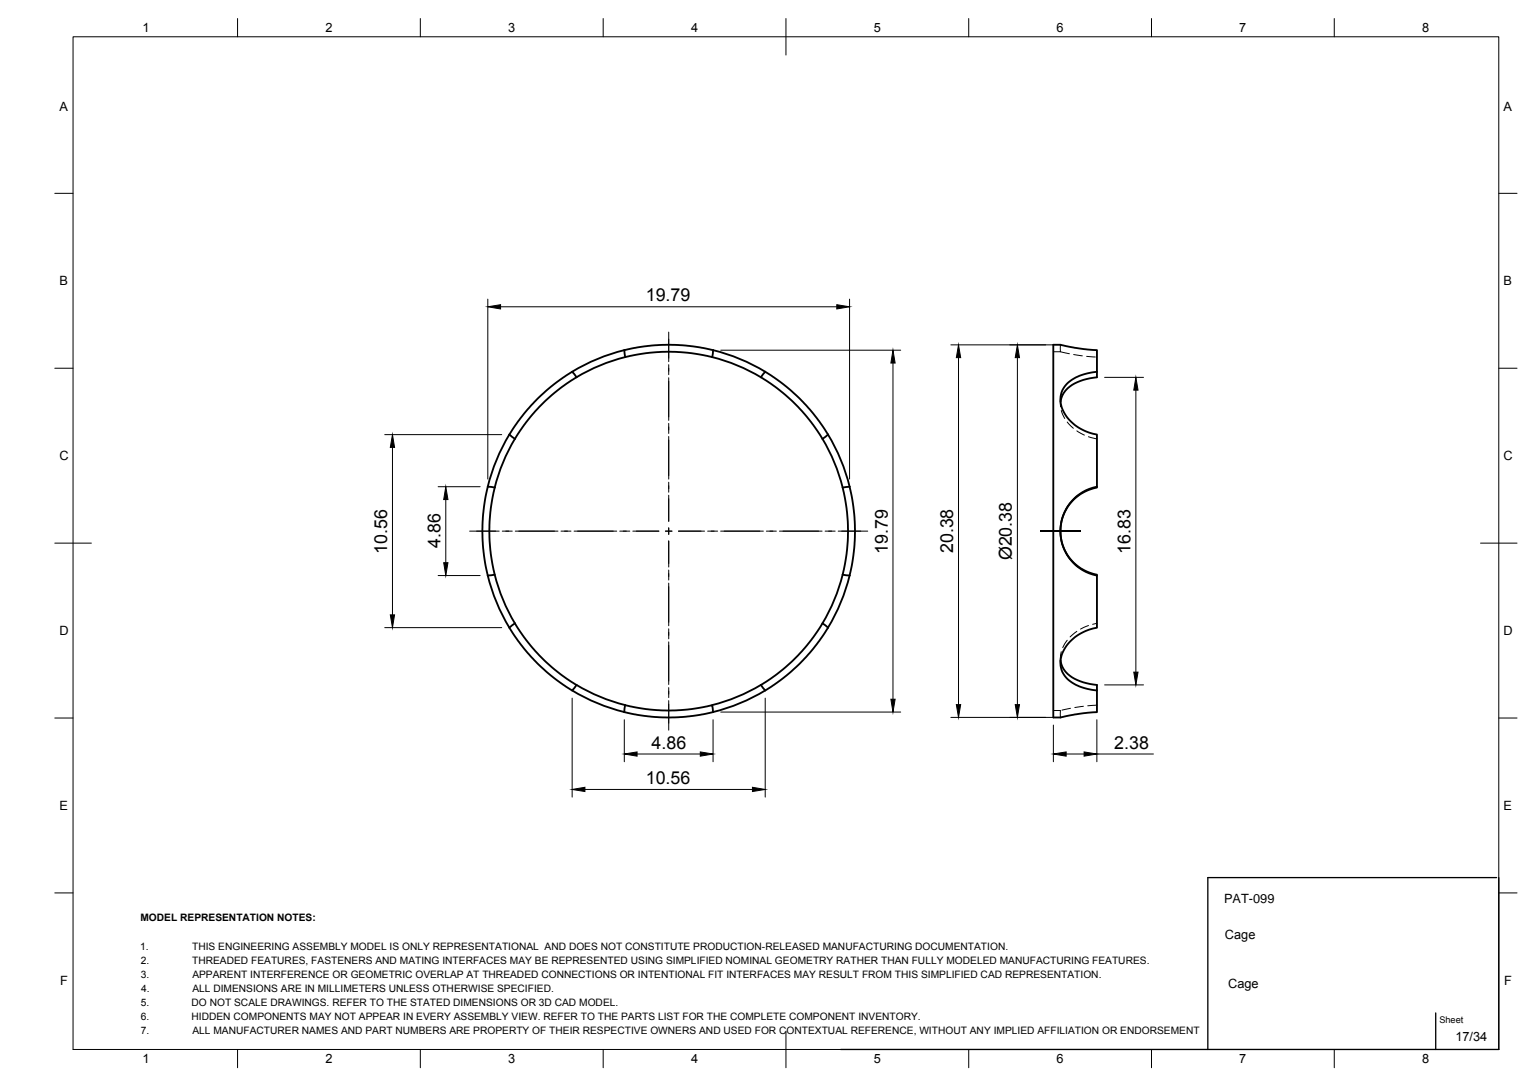
ISO-10303-21;
HEADER;
/* Generated by software containing ST-Developer
 * from STEP Tools, Inc. (www.steptools.com) 
 */

FILE_DESCRIPTION(
/* description */ ('PAT-099'),
/* implementation_level */ '2;1');

FILE_NAME(
/* name */ 'Cage.step',
/* time_stamp */ '2026-10-29T17:25:42-07:00',
/* author */ (''),
/* organization */ (''),
/* preprocessor_version */ 'ST-DEVELOPER v20.2',
/* originating_system */ 'Autodesk Translation Framework v15.17.0.0',
/* authorisation */ '');

FILE_SCHEMA (('AUTOMOTIVE_DESIGN { 1 0 10303 214 3 1 1 }'));
ENDSEC;

DATA;
#10=MECHANICAL_DESIGN_GEOMETRIC_PRESENTATION_REPRESENTATION('',(#367),#11035);
#19=SPHERICAL_SURFACE('',#5561,0.247676);
#20=SPHERICAL_SURFACE('',#5577,0.247676);
#21=SPHERICAL_SURFACE('',#5582,0.247676);
#22=SPHERICAL_SURFACE('',#5587,0.247676);
#23=SPHERICAL_SURFACE('',#5592,0.247676);
#24=SPHERICAL_SURFACE('',#5597,0.247676);
#25=SPHERICAL_SURFACE('',#5602,0.247676);
#26=SPHERICAL_SURFACE('',#5610,0.247676);
#269=B_SPLINE_CURVE_WITH_KNOTS('',3,(#10460,#10461,#10462,#10463,#10464,
#10465,#10466,#10467,#10468,#10469,#10470,#10471,#10472,#10473,#10474,#10475,
#10476,#10477,#10478,#10479,#10480,#10481),.UNSPECIFIED.,.F.,.F.,(4,2,2,
2,2,2,2,2,2,2,4),(0.0473477652366656,0.126350602536658,0.189525903804987,
0.252701205073317,0.313298422430275,0.373895639787233,0.434492857144191,
0.495090074501149,0.558265375769478,0.621440677037807,0.7004435143378),
 .UNSPECIFIED.);
#270=B_SPLINE_CURVE_WITH_KNOTS('',3,(#10485,#10486,#10487,#10488,#10489,
#10490,#10491,#10492,#10493,#10494,#10495,#10496,#10497,#10498,#10499,#10500,
#10501,#10502,#10503,#10504,#10505,#10506),.UNSPECIFIED.,.F.,.F.,(4,2,2,
2,2,2,2,2,2,2,4),(0.0464897534940957,0.0852567806515119,0.170513561303024,
0.246687263103517,0.308657850341199,0.370628437578881,0.432599024816563,
0.494569612054245,0.570743313854739,0.656000094506251,0.694767121663666),
 .UNSPECIFIED.);
#271=B_SPLINE_CURVE_WITH_KNOTS('',3,(#10512,#10513,#10514,#10515,#10516,
#10517,#10518,#10519,#10520,#10521,#10522,#10523,#10524,#10525,#10526,#10527,
#10528,#10529,#10530,#10531,#10532,#10533),.UNSPECIFIED.,.F.,.F.,(4,2,2,
2,2,2,2,2,2,2,4),(0.0464897534940957,0.0852567806515118,0.170513561303024,
0.246687263103517,0.308657850341199,0.370628437578881,0.432599024816563,
0.494569612054245,0.570743313854738,0.65600009450625,0.694767121663666),
 .UNSPECIFIED.);
#272=B_SPLINE_CURVE_WITH_KNOTS('',3,(#10537,#10538,#10539,#10540,#10541,
#10542,#10543,#10544,#10545,#10546,#10547,#10548,#10549,#10550,#10551,#10552,
#10553,#10554,#10555,#10556,#10557,#10558),.UNSPECIFIED.,.F.,.F.,(4,2,2,
2,2,2,2,2,2,2,4),(0.0464897534940957,0.0852567806515119,0.170513561303024,
0.246687263103517,0.308657850341199,0.370628437578881,0.432599024816563,
0.494569612054245,0.570743313854739,0.656000094506251,0.694767121663666),
 .UNSPECIFIED.);
#273=B_SPLINE_CURVE_WITH_KNOTS('',3,(#10562,#10563,#10564,#10565,#10566,
#10567,#10568,#10569,#10570,#10571,#10572,#10573),.UNSPECIFIED.,.F.,.F.,
(4,2,2,2,2,4),(0.0464897534940957,0.0852567806515119,0.170513561303024,
0.246687263103517,0.308657850341199,0.370628437578881),.UNSPECIFIED.);
#274=B_SPLINE_CURVE_WITH_KNOTS('',3,(#10578,#10579,#10580,#10581,#10582,
#10583,#10584,#10585,#10586,#10587,#10588,#10589),.UNSPECIFIED.,.F.,.F.,
(4,2,2,2,2,4),(0.370628437578881,0.432599024816563,0.494569612054245,0.570743313854738,
0.65600009450625,0.694767121663666),.UNSPECIFIED.);
#275=B_SPLINE_CURVE_WITH_KNOTS('',3,(#10593,#10594,#10595,#10596,#10597,
#10598,#10599,#10600,#10601,#10602,#10603,#10604,#10605,#10606,#10607,#10608,
#10609,#10610,#10611,#10612,#10613,#10614),.UNSPECIFIED.,.F.,.F.,(4,2,2,
2,2,2,2,2,2,2,4),(0.0464897534940957,0.0852567806515121,0.170513561303024,
0.246687263103518,0.308657850341199,0.370628437578881,0.432599024816563,
0.494569612054245,0.570743313854738,0.65600009450625,0.694767121663666),
 .UNSPECIFIED.);
#276=B_SPLINE_CURVE_WITH_KNOTS('',3,(#10618,#10619,#10620,#10621,#10622,
#10623,#10624,#10625,#10626,#10627,#10628,#10629,#10630,#10631,#10632,#10633,
#10634,#10635,#10636,#10637,#10638,#10639),.UNSPECIFIED.,.F.,.F.,(4,2,2,
2,2,2,2,2,2,2,4),(0.0464897534940957,0.0852567806515119,0.170513561303024,
0.246687263103517,0.308657850341199,0.370628437578881,0.432599024816563,
0.494569612054245,0.570743313854738,0.65600009450625,0.694767121663667),
 .UNSPECIFIED.);
#277=B_SPLINE_CURVE_WITH_KNOTS('',3,(#10643,#10644,#10645,#10646,#10647,
#10648,#10649,#10650,#10651,#10652,#10653,#10654,#10655,#10656,#10657,#10658,
#10659,#10660,#10661,#10662,#10663,#10664),.UNSPECIFIED.,.F.,.F.,(4,2,2,
2,2,2,2,2,2,2,4),(0.0464897534940957,0.0852567806515119,0.170513561303024,
0.246687263103517,0.308657850341199,0.370628437578881,0.432599024816563,
0.494569612054245,0.570743313854738,0.65600009450625,0.694767121663666),
 .UNSPECIFIED.);
#278=B_SPLINE_CURVE_WITH_KNOTS('',3,(#10668,#10669,#10670,#10671,#10672,
#10673,#10674,#10675,#10676,#10677,#10678,#10679,#10680,#10681,#10682,#10683,
#10684,#10685,#10686,#10687,#10688,#10689),.UNSPECIFIED.,.F.,.F.,(4,2,2,
2,2,2,2,2,2,2,4),(0.0464897534940957,0.0852567806515119,0.170513561303024,
0.246687263103517,0.308657850341199,0.370628437578881,0.432599024816563,
0.494569612054245,0.570743313854739,0.656000094506251,0.694767121663667),
 .UNSPECIFIED.);
#279=B_SPLINE_CURVE_WITH_KNOTS('',3,(#10697,#10698,#10699,#10700,#10701,
#10702,#10703,#10704,#10705,#10706,#10707,#10708,#10709,#10710,#10711,#10712,
#10713,#10714,#10715,#10716,#10717,#10718),.UNSPECIFIED.,.F.,.F.,(4,2,2,
2,2,2,2,2,2,2,4),(0.0473477652366656,0.126350602536658,0.189525903804987,
0.252701205073316,0.313298422430274,0.373895639787232,0.434492857144191,
0.495090074501149,0.558265375769478,0.621440677037807,0.7004435143378),
 .UNSPECIFIED.);
#280=B_SPLINE_CURVE_WITH_KNOTS('',3,(#10726,#10727,#10728,#10729,#10730,
#10731,#10732,#10733,#10734,#10735,#10736,#10737,#10738,#10739,#10740,#10741,
#10742,#10743,#10744,#10745,#10746,#10747),.UNSPECIFIED.,.F.,.F.,(4,2,2,
2,2,2,2,2,2,2,4),(0.0473477652366656,0.126350602536658,0.189525903804987,
0.252701205073317,0.313298422430275,0.373895639787233,0.434492857144191,
0.495090074501149,0.558265375769478,0.621440677037807,0.7004435143378),
 .UNSPECIFIED.);
#281=B_SPLINE_CURVE_WITH_KNOTS('',3,(#10756,#10757,#10758,#10759,#10760,
#10761,#10762,#10763,#10764,#10765,#10766,#10767),.UNSPECIFIED.,.F.,.F.,
(4,2,2,2,2,4),(0.0473477652366656,0.126350602536658,0.189525903804987,0.252701205073316,
0.313298422430275,0.373895639787233),.UNSPECIFIED.);
#282=B_SPLINE_CURVE_WITH_KNOTS('',3,(#10769,#10770,#10771,#10772,#10773,
#10774,#10775,#10776,#10777,#10778,#10779,#10780),.UNSPECIFIED.,.F.,.F.,
(4,2,2,2,2,4),(0.373895639787233,0.434492857144191,0.495090074501149,0.558265375769478,
0.621440677037807,0.7004435143378),.UNSPECIFIED.);
#283=B_SPLINE_CURVE_WITH_KNOTS('',3,(#10787,#10788,#10789,#10790,#10791,
#10792,#10793,#10794,#10795,#10796,#10797,#10798,#10799,#10800,#10801,#10802,
#10803,#10804,#10805,#10806,#10807,#10808),.UNSPECIFIED.,.F.,.F.,(4,2,2,
2,2,2,2,2,2,2,4),(0.0473477652366656,0.126350602536658,0.189525903804987,
0.252701205073316,0.313298422430275,0.373895639787233,0.434492857144191,
0.495090074501149,0.558265375769478,0.621440677037807,0.7004435143378),
 .UNSPECIFIED.);
#284=B_SPLINE_CURVE_WITH_KNOTS('',3,(#10816,#10817,#10818,#10819,#10820,
#10821,#10822,#10823,#10824,#10825,#10826,#10827,#10828,#10829,#10830,#10831,
#10832,#10833,#10834,#10835,#10836,#10837),.UNSPECIFIED.,.F.,.F.,(4,2,2,
2,2,2,2,2,2,2,4),(0.0473477652366656,0.126350602536658,0.189525903804987,
0.252701205073317,0.313298422430275,0.373895639787233,0.434492857144191,
0.495090074501149,0.558265375769478,0.621440677037807,0.7004435143378),
 .UNSPECIFIED.);
#285=B_SPLINE_CURVE_WITH_KNOTS('',3,(#10845,#10846,#10847,#10848,#10849,
#10850,#10851,#10852,#10853,#10854,#10855,#10856,#10857,#10858,#10859,#10860,
#10861,#10862,#10863,#10864,#10865,#10866),.UNSPECIFIED.,.F.,.F.,(4,2,2,
2,2,2,2,2,2,2,4),(0.0473477652366656,0.126350602536658,0.189525903804987,
0.252701205073316,0.313298422430275,0.373895639787233,0.434492857144191,
0.495090074501149,0.558265375769478,0.621440677037807,0.7004435143378),
 .UNSPECIFIED.);
#286=B_SPLINE_CURVE_WITH_KNOTS('',3,(#10875,#10876,#10877,#10878,#10879,
#10880,#10881,#10882,#10883,#10884,#10885,#10886,#10887,#10888,#10889,#10890,
#10891,#10892,#10893,#10894,#10895,#10896),.UNSPECIFIED.,.F.,.F.,(4,2,2,
2,2,2,2,2,2,2,4),(0.0473477652366656,0.126350602536658,0.189525903804987,
0.252701205073317,0.313298422430275,0.373895639787233,0.434492857144191,
0.495090074501149,0.558265375769478,0.621440677037807,0.7004435143378),
 .UNSPECIFIED.);
#310=SHAPE_REPRESENTATION_RELATIONSHIP('SRR','None',#11183,#335);
#335=ADVANCED_BREP_SHAPE_REPRESENTATION('',(#398),#11033);
#367=STYLED_ITEM('',(#11386),#398);
#398=MANIFOLD_SOLID_BREP('Continuous crown cage',#4737);
#518=FACE_BOUND('',#1329,.T.);
#646=PLANE('',#5574);
#647=PLANE('',#5579);
#648=PLANE('',#5584);
#649=PLANE('',#5589);
#650=PLANE('',#5594);
#651=PLANE('',#5599);
#652=PLANE('',#5608);
#653=PLANE('',#5612);
#654=PLANE('',#5613);
#913=FACE_OUTER_BOUND('',#1311,.T.);
#914=FACE_OUTER_BOUND('',#1312,.T.);
#915=FACE_OUTER_BOUND('',#1313,.T.);
#916=FACE_OUTER_BOUND('',#1314,.T.);
#917=FACE_OUTER_BOUND('',#1315,.T.);
#918=FACE_OUTER_BOUND('',#1316,.T.);
#919=FACE_OUTER_BOUND('',#1317,.T.);
#920=FACE_OUTER_BOUND('',#1318,.T.);
#921=FACE_OUTER_BOUND('',#1319,.T.);
#922=FACE_OUTER_BOUND('',#1320,.T.);
#923=FACE_OUTER_BOUND('',#1321,.T.);
#924=FACE_OUTER_BOUND('',#1322,.T.);
#925=FACE_OUTER_BOUND('',#1323,.T.);
#926=FACE_OUTER_BOUND('',#1324,.T.);
#927=FACE_OUTER_BOUND('',#1325,.T.);
#928=FACE_OUTER_BOUND('',#1326,.T.);
#929=FACE_OUTER_BOUND('',#1327,.T.);
#930=FACE_OUTER_BOUND('',#1328,.T.);
#931=FACE_OUTER_BOUND('',#1330,.T.);
#1311=EDGE_LOOP('',(#4177,#4178,#4179,#4180));
#1312=EDGE_LOOP('',(#4181,#4182,#4183,#4184,#4185,#4186,#4187,#4188,#4189,
#4190,#4191,#4192,#4193,#4194,#4195,#4196,#4197,#4198,#4199,#4200));
#1313=EDGE_LOOP('',(#4201,#4202,#4203,#4204));
#1314=EDGE_LOOP('',(#4205,#4206,#4207,#4208));
#1315=EDGE_LOOP('',(#4209,#4210,#4211,#4212));
#1316=EDGE_LOOP('',(#4213,#4214,#4215,#4216));
#1317=EDGE_LOOP('',(#4217,#4218,#4219,#4220));
#1318=EDGE_LOOP('',(#4221,#4222,#4223,#4224,#4225,#4226));
#1319=EDGE_LOOP('',(#4227,#4228,#4229,#4230));
#1320=EDGE_LOOP('',(#4231,#4232,#4233,#4234));
#1321=EDGE_LOOP('',(#4235,#4236,#4237,#4238));
#1322=EDGE_LOOP('',(#4239,#4240,#4241,#4242));
#1323=EDGE_LOOP('',(#4243,#4244,#4245,#4246));
#1324=EDGE_LOOP('',(#4247,#4248,#4249,#4250));
#1325=EDGE_LOOP('',(#4251,#4252,#4253,#4254,#4255,#4256,#4257,#4258,#4259,
#4260,#4261,#4262,#4263,#4264,#4265,#4266,#4267,#4268,#4269,#4270));
#1326=EDGE_LOOP('',(#4271,#4272,#4273,#4274));
#1327=EDGE_LOOP('',(#4275,#4276,#4277,#4278));
#1328=EDGE_LOOP('',(#4279));
#1329=EDGE_LOOP('',(#4280));
#1330=EDGE_LOOP('',(#4281,#4282,#4283,#4284));
#1589=LINE('',#10575,#1841);
#1590=LINE('',#10871,#1842);
#1841=VECTOR('',#7018,1.019052);
#1842=VECTOR('',#7095,0.980948);
#2096=CIRCLE('',#5562,0.243053047864041);
#2097=CIRCLE('',#5563,0.243053047864041);
#2098=CIRCLE('',#5565,1.019052);
#2099=CIRCLE('',#5566,1.019052);
#2100=CIRCLE('',#5567,1.019052);
#2101=CIRCLE('',#5568,1.019052);
#2102=CIRCLE('',#5569,1.019052);
#2103=CIRCLE('',#5570,1.019052);
#2104=CIRCLE('',#5571,1.019052);
#2105=CIRCLE('',#5572,1.019052);
#2106=CIRCLE('',#5573,1.019052);
#2107=CIRCLE('',#5575,0.980948);
#2108=CIRCLE('',#5576,0.243053047864041);
#2109=CIRCLE('',#5578,0.243053047864041);
#2110=CIRCLE('',#5580,0.980948);
#2111=CIRCLE('',#5581,0.243053047864041);
#2112=CIRCLE('',#5583,0.243053047864041);
#2113=CIRCLE('',#5585,0.980948);
#2114=CIRCLE('',#5586,0.243053047864041);
#2115=CIRCLE('',#5588,0.243053047864041);
#2116=CIRCLE('',#5590,0.980948);
#2117=CIRCLE('',#5591,0.243053047864041);
#2118=CIRCLE('',#5593,0.243053047864041);
#2119=CIRCLE('',#5595,0.980948);
#2120=CIRCLE('',#5596,0.243053047864041);
#2121=CIRCLE('',#5598,0.243053047864041);
#2122=CIRCLE('',#5600,0.980948);
#2123=CIRCLE('',#5601,0.243053047864041);
#2124=CIRCLE('',#5603,0.243053047864041);
#2125=CIRCLE('',#5605,0.980948);
#2126=CIRCLE('',#5606,0.980948);
#2127=CIRCLE('',#5607,0.980948);
#2128=CIRCLE('',#5609,0.243053047864041);
#2129=CIRCLE('',#5611,0.243053047864041);
#2498=VERTEX_POINT('',#10458);
#2499=VERTEX_POINT('',#10459);
#2500=VERTEX_POINT('',#10482);
#2501=VERTEX_POINT('',#10484);
#2502=VERTEX_POINT('',#10509);
#2503=VERTEX_POINT('',#10511);
#2504=VERTEX_POINT('',#10534);
#2505=VERTEX_POINT('',#10536);
#2506=VERTEX_POINT('',#10559);
#2507=VERTEX_POINT('',#10561);
#2508=VERTEX_POINT('',#10574);
#2509=VERTEX_POINT('',#10577);
#2510=VERTEX_POINT('',#10590);
#2511=VERTEX_POINT('',#10592);
#2512=VERTEX_POINT('',#10615);
#2513=VERTEX_POINT('',#10617);
#2514=VERTEX_POINT('',#10640);
#2515=VERTEX_POINT('',#10642);
#2516=VERTEX_POINT('',#10665);
#2517=VERTEX_POINT('',#10667);
#2518=VERTEX_POINT('',#10692);
#2519=VERTEX_POINT('',#10696);
#2520=VERTEX_POINT('',#10721);
#2521=VERTEX_POINT('',#10725);
#2522=VERTEX_POINT('',#10750);
#2523=VERTEX_POINT('',#10754);
#2524=VERTEX_POINT('',#10755);
#2525=VERTEX_POINT('',#10782);
#2526=VERTEX_POINT('',#10786);
#2527=VERTEX_POINT('',#10811);
#2528=VERTEX_POINT('',#10815);
#2529=VERTEX_POINT('',#10840);
#2530=VERTEX_POINT('',#10844);
#2531=VERTEX_POINT('',#10869);
#2532=VERTEX_POINT('',#10872);
#2533=VERTEX_POINT('',#10874);
#3065=EDGE_CURVE('',#2498,#2499,#269,.T.);
#3066=EDGE_CURVE('',#2500,#2498,#2096,.T.);
#3067=EDGE_CURVE('',#2501,#2500,#270,.T.);
#3068=EDGE_CURVE('',#2499,#2501,#2097,.T.);
#3069=EDGE_CURVE('',#2502,#2500,#2098,.T.);
#3070=EDGE_CURVE('',#2502,#2503,#271,.T.);
#3071=EDGE_CURVE('',#2504,#2503,#2099,.T.);
#3072=EDGE_CURVE('',#2504,#2505,#272,.T.);
#3073=EDGE_CURVE('',#2506,#2505,#2100,.T.);
#3074=EDGE_CURVE('',#2506,#2507,#273,.T.);
#3075=EDGE_CURVE('',#2507,#2508,#1589,.T.);
#3076=EDGE_CURVE('',#2508,#2508,#2101,.T.);
#3077=EDGE_CURVE('',#2507,#2509,#274,.T.);
#3078=EDGE_CURVE('',#2510,#2509,#2102,.T.);
#3079=EDGE_CURVE('',#2510,#2511,#275,.T.);
#3080=EDGE_CURVE('',#2512,#2511,#2103,.T.);
#3081=EDGE_CURVE('',#2512,#2513,#276,.T.);
#3082=EDGE_CURVE('',#2514,#2513,#2104,.T.);
#3083=EDGE_CURVE('',#2514,#2515,#277,.T.);
#3084=EDGE_CURVE('',#2516,#2515,#2105,.T.);
#3085=EDGE_CURVE('',#2516,#2517,#278,.T.);
#3086=EDGE_CURVE('',#2501,#2517,#2106,.T.);
#3087=EDGE_CURVE('',#2498,#2518,#2107,.T.);
#3088=EDGE_CURVE('',#2518,#2502,#2108,.T.);
#3089=EDGE_CURVE('',#2519,#2518,#279,.T.);
#3090=EDGE_CURVE('',#2503,#2519,#2109,.T.);
#3091=EDGE_CURVE('',#2519,#2520,#2110,.T.);
#3092=EDGE_CURVE('',#2520,#2504,#2111,.T.);
#3093=EDGE_CURVE('',#2521,#2520,#280,.T.);
#3094=EDGE_CURVE('',#2505,#2521,#2112,.T.);
#3095=EDGE_CURVE('',#2521,#2522,#2113,.T.);
#3096=EDGE_CURVE('',#2522,#2506,#2114,.T.);
#3097=EDGE_CURVE('',#2523,#2524,#281,.T.);
#3098=EDGE_CURVE('',#2509,#2523,#2115,.T.);
#3099=EDGE_CURVE('',#2524,#2522,#282,.T.);
#3100=EDGE_CURVE('',#2523,#2525,#2116,.T.);
#3101=EDGE_CURVE('',#2525,#2510,#2117,.T.);
#3102=EDGE_CURVE('',#2526,#2525,#283,.T.);
#3103=EDGE_CURVE('',#2511,#2526,#2118,.T.);
#3104=EDGE_CURVE('',#2526,#2527,#2119,.T.);
#3105=EDGE_CURVE('',#2527,#2512,#2120,.T.);
#3106=EDGE_CURVE('',#2528,#2527,#284,.T.);
#3107=EDGE_CURVE('',#2513,#2528,#2121,.T.);
#3108=EDGE_CURVE('',#2528,#2529,#2122,.T.);
#3109=EDGE_CURVE('',#2529,#2514,#2123,.T.);
#3110=EDGE_CURVE('',#2530,#2529,#285,.T.);
#3111=EDGE_CURVE('',#2515,#2530,#2124,.T.);
#3112=EDGE_CURVE('',#2531,#2531,#2125,.T.);
#3113=EDGE_CURVE('',#2531,#2524,#1590,.T.);
#3114=EDGE_CURVE('',#2532,#2499,#2126,.T.);
#3115=EDGE_CURVE('',#2532,#2533,#286,.T.);
#3116=EDGE_CURVE('',#2530,#2533,#2127,.T.);
#3117=EDGE_CURVE('',#2517,#2532,#2128,.T.);
#3118=EDGE_CURVE('',#2533,#2516,#2129,.T.);
#4177=ORIENTED_EDGE('',*,*,#3065,.F.);
#4178=ORIENTED_EDGE('',*,*,#3066,.F.);
#4179=ORIENTED_EDGE('',*,*,#3067,.F.);
#4180=ORIENTED_EDGE('',*,*,#3068,.F.);
#4181=ORIENTED_EDGE('',*,*,#3067,.T.);
#4182=ORIENTED_EDGE('',*,*,#3069,.F.);
#4183=ORIENTED_EDGE('',*,*,#3070,.T.);
#4184=ORIENTED_EDGE('',*,*,#3071,.F.);
#4185=ORIENTED_EDGE('',*,*,#3072,.T.);
#4186=ORIENTED_EDGE('',*,*,#3073,.F.);
#4187=ORIENTED_EDGE('',*,*,#3074,.T.);
#4188=ORIENTED_EDGE('',*,*,#3075,.T.);
#4189=ORIENTED_EDGE('',*,*,#3076,.F.);
#4190=ORIENTED_EDGE('',*,*,#3075,.F.);
#4191=ORIENTED_EDGE('',*,*,#3077,.T.);
#4192=ORIENTED_EDGE('',*,*,#3078,.F.);
#4193=ORIENTED_EDGE('',*,*,#3079,.T.);
#4194=ORIENTED_EDGE('',*,*,#3080,.F.);
#4195=ORIENTED_EDGE('',*,*,#3081,.T.);
#4196=ORIENTED_EDGE('',*,*,#3082,.F.);
#4197=ORIENTED_EDGE('',*,*,#3083,.T.);
#4198=ORIENTED_EDGE('',*,*,#3084,.F.);
#4199=ORIENTED_EDGE('',*,*,#3085,.T.);
#4200=ORIENTED_EDGE('',*,*,#3086,.F.);
#4201=ORIENTED_EDGE('',*,*,#3066,.T.);
#4202=ORIENTED_EDGE('',*,*,#3087,.T.);
#4203=ORIENTED_EDGE('',*,*,#3088,.T.);
#4204=ORIENTED_EDGE('',*,*,#3069,.T.);
#4205=ORIENTED_EDGE('',*,*,#3089,.F.);
#4206=ORIENTED_EDGE('',*,*,#3090,.F.);
#4207=ORIENTED_EDGE('',*,*,#3070,.F.);
#4208=ORIENTED_EDGE('',*,*,#3088,.F.);
#4209=ORIENTED_EDGE('',*,*,#3090,.T.);
#4210=ORIENTED_EDGE('',*,*,#3091,.T.);
#4211=ORIENTED_EDGE('',*,*,#3092,.T.);
#4212=ORIENTED_EDGE('',*,*,#3071,.T.);
#4213=ORIENTED_EDGE('',*,*,#3093,.F.);
#4214=ORIENTED_EDGE('',*,*,#3094,.F.);
#4215=ORIENTED_EDGE('',*,*,#3072,.F.);
#4216=ORIENTED_EDGE('',*,*,#3092,.F.);
#4217=ORIENTED_EDGE('',*,*,#3094,.T.);
#4218=ORIENTED_EDGE('',*,*,#3095,.T.);
#4219=ORIENTED_EDGE('',*,*,#3096,.T.);
#4220=ORIENTED_EDGE('',*,*,#3073,.T.);
#4221=ORIENTED_EDGE('',*,*,#3097,.F.);
#4222=ORIENTED_EDGE('',*,*,#3098,.F.);
#4223=ORIENTED_EDGE('',*,*,#3077,.F.);
#4224=ORIENTED_EDGE('',*,*,#3074,.F.);
#4225=ORIENTED_EDGE('',*,*,#3096,.F.);
#4226=ORIENTED_EDGE('',*,*,#3099,.F.);
#4227=ORIENTED_EDGE('',*,*,#3098,.T.);
#4228=ORIENTED_EDGE('',*,*,#3100,.T.);
#4229=ORIENTED_EDGE('',*,*,#3101,.T.);
#4230=ORIENTED_EDGE('',*,*,#3078,.T.);
#4231=ORIENTED_EDGE('',*,*,#3102,.F.);
#4232=ORIENTED_EDGE('',*,*,#3103,.F.);
#4233=ORIENTED_EDGE('',*,*,#3079,.F.);
#4234=ORIENTED_EDGE('',*,*,#3101,.F.);
#4235=ORIENTED_EDGE('',*,*,#3103,.T.);
#4236=ORIENTED_EDGE('',*,*,#3104,.T.);
#4237=ORIENTED_EDGE('',*,*,#3105,.T.);
#4238=ORIENTED_EDGE('',*,*,#3080,.T.);
#4239=ORIENTED_EDGE('',*,*,#3106,.F.);
#4240=ORIENTED_EDGE('',*,*,#3107,.F.);
#4241=ORIENTED_EDGE('',*,*,#3081,.F.);
#4242=ORIENTED_EDGE('',*,*,#3105,.F.);
#4243=ORIENTED_EDGE('',*,*,#3107,.T.);
#4244=ORIENTED_EDGE('',*,*,#3108,.T.);
#4245=ORIENTED_EDGE('',*,*,#3109,.T.);
#4246=ORIENTED_EDGE('',*,*,#3082,.T.);
#4247=ORIENTED_EDGE('',*,*,#3083,.F.);
#4248=ORIENTED_EDGE('',*,*,#3109,.F.);
#4249=ORIENTED_EDGE('',*,*,#3110,.F.);
#4250=ORIENTED_EDGE('',*,*,#3111,.F.);
#4251=ORIENTED_EDGE('',*,*,#3112,.F.);
#4252=ORIENTED_EDGE('',*,*,#3113,.T.);
#4253=ORIENTED_EDGE('',*,*,#3099,.T.);
#4254=ORIENTED_EDGE('',*,*,#3095,.F.);
#4255=ORIENTED_EDGE('',*,*,#3093,.T.);
#4256=ORIENTED_EDGE('',*,*,#3091,.F.);
#4257=ORIENTED_EDGE('',*,*,#3089,.T.);
#4258=ORIENTED_EDGE('',*,*,#3087,.F.);
#4259=ORIENTED_EDGE('',*,*,#3065,.T.);
#4260=ORIENTED_EDGE('',*,*,#3114,.F.);
#4261=ORIENTED_EDGE('',*,*,#3115,.T.);
#4262=ORIENTED_EDGE('',*,*,#3116,.F.);
#4263=ORIENTED_EDGE('',*,*,#3110,.T.);
#4264=ORIENTED_EDGE('',*,*,#3108,.F.);
#4265=ORIENTED_EDGE('',*,*,#3106,.T.);
#4266=ORIENTED_EDGE('',*,*,#3104,.F.);
#4267=ORIENTED_EDGE('',*,*,#3102,.T.);
#4268=ORIENTED_EDGE('',*,*,#3100,.F.);
#4269=ORIENTED_EDGE('',*,*,#3097,.T.);
#4270=ORIENTED_EDGE('',*,*,#3113,.F.);
#4271=ORIENTED_EDGE('',*,*,#3068,.T.);
#4272=ORIENTED_EDGE('',*,*,#3086,.T.);
#4273=ORIENTED_EDGE('',*,*,#3117,.T.);
#4274=ORIENTED_EDGE('',*,*,#3114,.T.);
#4275=ORIENTED_EDGE('',*,*,#3085,.F.);
#4276=ORIENTED_EDGE('',*,*,#3118,.F.);
#4277=ORIENTED_EDGE('',*,*,#3115,.F.);
#4278=ORIENTED_EDGE('',*,*,#3117,.F.);
#4279=ORIENTED_EDGE('',*,*,#3076,.T.);
#4280=ORIENTED_EDGE('',*,*,#3112,.T.);
#4281=ORIENTED_EDGE('',*,*,#3111,.T.);
#4282=ORIENTED_EDGE('',*,*,#3116,.T.);
#4283=ORIENTED_EDGE('',*,*,#3118,.T.);
#4284=ORIENTED_EDGE('',*,*,#3084,.T.);
#4418=CYLINDRICAL_SURFACE('',#5564,1.019052);
#4419=CYLINDRICAL_SURFACE('',#5604,0.980948);
#4678=ADVANCED_FACE('',(#913),#19,.F.);
#4679=ADVANCED_FACE('',(#914),#4418,.T.);
#4680=ADVANCED_FACE('',(#915),#646,.T.);
#4681=ADVANCED_FACE('',(#916),#20,.F.);
#4682=ADVANCED_FACE('',(#917),#647,.T.);
#4683=ADVANCED_FACE('',(#918),#21,.F.);
#4684=ADVANCED_FACE('',(#919),#648,.T.);
#4685=ADVANCED_FACE('',(#920),#22,.F.);
#4686=ADVANCED_FACE('',(#921),#649,.T.);
#4687=ADVANCED_FACE('',(#922),#23,.F.);
#4688=ADVANCED_FACE('',(#923),#650,.T.);
#4689=ADVANCED_FACE('',(#924),#24,.F.);
#4690=ADVANCED_FACE('',(#925),#651,.T.);
#4691=ADVANCED_FACE('',(#926),#25,.F.);
#4692=ADVANCED_FACE('',(#927),#4419,.F.);
#4693=ADVANCED_FACE('',(#928),#652,.T.);
#4694=ADVANCED_FACE('',(#929),#26,.F.);
#4695=ADVANCED_FACE('',(#930,#518),#653,.T.);
#4696=ADVANCED_FACE('',(#931),#654,.T.);
#4737=CLOSED_SHELL('',(#4678,#4679,#4680,#4681,#4682,#4683,#4684,#4685,
#4686,#4687,#4688,#4689,#4690,#4691,#4692,#4693,#4694,#4695,#4696));
#5560=AXIS2_PLACEMENT_3D('',#10456,#7002,#7003);
#5561=AXIS2_PLACEMENT_3D('',#10457,#7004,#7005);
#5562=AXIS2_PLACEMENT_3D('',#10483,#7006,#7007);
#5563=AXIS2_PLACEMENT_3D('',#10507,#7008,#7009);
#5564=AXIS2_PLACEMENT_3D('',#10508,#7010,#7011);
#5565=AXIS2_PLACEMENT_3D('',#10510,#7012,#7013);
#5566=AXIS2_PLACEMENT_3D('',#10535,#7014,#7015);
#5567=AXIS2_PLACEMENT_3D('',#10560,#7016,#7017);
#5568=AXIS2_PLACEMENT_3D('',#10576,#7019,#7020);
#5569=AXIS2_PLACEMENT_3D('',#10591,#7021,#7022);
#5570=AXIS2_PLACEMENT_3D('',#10616,#7023,#7024);
#5571=AXIS2_PLACEMENT_3D('',#10641,#7025,#7026);
#5572=AXIS2_PLACEMENT_3D('',#10666,#7027,#7028);
#5573=AXIS2_PLACEMENT_3D('',#10690,#7029,#7030);
#5574=AXIS2_PLACEMENT_3D('',#10691,#7031,#7032);
#5575=AXIS2_PLACEMENT_3D('',#10693,#7033,#7034);
#5576=AXIS2_PLACEMENT_3D('',#10694,#7035,#7036);
#5577=AXIS2_PLACEMENT_3D('',#10695,#7037,#7038);
#5578=AXIS2_PLACEMENT_3D('',#10719,#7039,#7040);
#5579=AXIS2_PLACEMENT_3D('',#10720,#7041,#7042);
#5580=AXIS2_PLACEMENT_3D('',#10722,#7043,#7044);
#5581=AXIS2_PLACEMENT_3D('',#10723,#7045,#7046);
#5582=AXIS2_PLACEMENT_3D('',#10724,#7047,#7048);
#5583=AXIS2_PLACEMENT_3D('',#10748,#7049,#7050);
#5584=AXIS2_PLACEMENT_3D('',#10749,#7051,#7052);
#5585=AXIS2_PLACEMENT_3D('',#10751,#7053,#7054);
#5586=AXIS2_PLACEMENT_3D('',#10752,#7055,#7056);
#5587=AXIS2_PLACEMENT_3D('',#10753,#7057,#7058);
#5588=AXIS2_PLACEMENT_3D('',#10768,#7059,#7060);
#5589=AXIS2_PLACEMENT_3D('',#10781,#7061,#7062);
#5590=AXIS2_PLACEMENT_3D('',#10783,#7063,#7064);
#5591=AXIS2_PLACEMENT_3D('',#10784,#7065,#7066);
#5592=AXIS2_PLACEMENT_3D('',#10785,#7067,#7068);
#5593=AXIS2_PLACEMENT_3D('',#10809,#7069,#7070);
#5594=AXIS2_PLACEMENT_3D('',#10810,#7071,#7072);
#5595=AXIS2_PLACEMENT_3D('',#10812,#7073,#7074);
#5596=AXIS2_PLACEMENT_3D('',#10813,#7075,#7076);
#5597=AXIS2_PLACEMENT_3D('',#10814,#7077,#7078);
#5598=AXIS2_PLACEMENT_3D('',#10838,#7079,#7080);
#5599=AXIS2_PLACEMENT_3D('',#10839,#7081,#7082);
#5600=AXIS2_PLACEMENT_3D('',#10841,#7083,#7084);
#5601=AXIS2_PLACEMENT_3D('',#10842,#7085,#7086);
#5602=AXIS2_PLACEMENT_3D('',#10843,#7087,#7088);
#5603=AXIS2_PLACEMENT_3D('',#10867,#7089,#7090);
#5604=AXIS2_PLACEMENT_3D('',#10868,#7091,#7092);
#5605=AXIS2_PLACEMENT_3D('',#10870,#7093,#7094);
#5606=AXIS2_PLACEMENT_3D('',#10873,#7096,#7097);
#5607=AXIS2_PLACEMENT_3D('',#10897,#7098,#7099);
#5608=AXIS2_PLACEMENT_3D('',#10898,#7100,#7101);
#5609=AXIS2_PLACEMENT_3D('',#10899,#7102,#7103);
#5610=AXIS2_PLACEMENT_3D('',#10900,#7104,#7105);
#5611=AXIS2_PLACEMENT_3D('',#10901,#7106,#7107);
#5612=AXIS2_PLACEMENT_3D('',#10902,#7108,#7109);
#5613=AXIS2_PLACEMENT_3D('',#10903,#7110,#7111);
#7002=DIRECTION('axis',(0.,0.,1.));
#7003=DIRECTION('refdir',(1.,0.,0.));
#7004=DIRECTION('center_axis',(0.,0.,1.));
#7005=DIRECTION('ref_axis',(1.,0.,0.));
#7006=DIRECTION('center_axis',(0.,-1.,0.));
#7007=DIRECTION('ref_axis',(0.,0.,-1.));
#7008=DIRECTION('center_axis',(0.,-1.,0.));
#7009=DIRECTION('ref_axis',(0.,0.,-1.));
#7010=DIRECTION('center_axis',(0.,1.,0.));
#7011=DIRECTION('ref_axis',(1.,0.,0.));
#7012=DIRECTION('center_axis',(0.,1.,0.));
#7013=DIRECTION('ref_axis',(1.,0.,0.));
#7014=DIRECTION('center_axis',(0.,1.,0.));
#7015=DIRECTION('ref_axis',(1.,0.,0.));
#7016=DIRECTION('center_axis',(0.,1.,0.));
#7017=DIRECTION('ref_axis',(1.,0.,0.));
#7018=DIRECTION('',(0.,-1.,0.));
#7019=DIRECTION('center_axis',(0.,-1.,0.));
#7020=DIRECTION('ref_axis',(1.,0.,0.));
#7021=DIRECTION('center_axis',(0.,1.,0.));
#7022=DIRECTION('ref_axis',(1.,0.,0.));
#7023=DIRECTION('center_axis',(0.,1.,0.));
#7024=DIRECTION('ref_axis',(1.,0.,0.));
#7025=DIRECTION('center_axis',(0.,1.,0.));
#7026=DIRECTION('ref_axis',(1.,0.,0.));
#7027=DIRECTION('center_axis',(0.,1.,0.));
#7028=DIRECTION('ref_axis',(1.,0.,0.));
#7029=DIRECTION('center_axis',(0.,1.,0.));
#7030=DIRECTION('ref_axis',(1.,0.,0.));
#7031=DIRECTION('center_axis',(0.,1.,0.));
#7032=DIRECTION('ref_axis',(1.,0.,0.));
#7033=DIRECTION('center_axis',(0.,-1.,0.));
#7034=DIRECTION('ref_axis',(1.,0.,0.));
#7035=DIRECTION('center_axis',(0.,-1.,0.));
#7036=DIRECTION('ref_axis',(0.,0.,-1.));
#7037=DIRECTION('center_axis',(6.12323399573677E-17,0.,1.));
#7038=DIRECTION('ref_axis',(1.,0.,0.));
#7039=DIRECTION('center_axis',(0.,-1.,0.));
#7040=DIRECTION('ref_axis',(0.,0.,-1.));
#7041=DIRECTION('center_axis',(0.,1.,0.));
#7042=DIRECTION('ref_axis',(1.,0.,0.));
#7043=DIRECTION('center_axis',(0.,-1.,0.));
#7044=DIRECTION('ref_axis',(1.,0.,0.));
#7045=DIRECTION('center_axis',(0.,-1.,0.));
#7046=DIRECTION('ref_axis',(0.,0.,-1.));
#7047=DIRECTION('center_axis',(0.,0.,1.));
#7048=DIRECTION('ref_axis',(1.,0.,0.));
#7049=DIRECTION('center_axis',(0.,-1.,0.));
#7050=DIRECTION('ref_axis',(0.,0.,-1.));
#7051=DIRECTION('center_axis',(0.,1.,0.));
#7052=DIRECTION('ref_axis',(1.,0.,0.));
#7053=DIRECTION('center_axis',(0.,-1.,0.));
#7054=DIRECTION('ref_axis',(1.,0.,0.));
#7055=DIRECTION('center_axis',(0.,-1.,0.));
#7056=DIRECTION('ref_axis',(0.,0.,-1.));
#7057=DIRECTION('center_axis',(0.,0.,1.));
#7058=DIRECTION('ref_axis',(1.,0.,0.));
#7059=DIRECTION('center_axis',(0.,-1.,0.));
#7060=DIRECTION('ref_axis',(0.,0.,-1.));
#7061=DIRECTION('center_axis',(0.,1.,0.));
#7062=DIRECTION('ref_axis',(1.,0.,0.));
#7063=DIRECTION('center_axis',(0.,-1.,0.));
#7064=DIRECTION('ref_axis',(1.,0.,0.));
#7065=DIRECTION('center_axis',(0.,-1.,0.));
#7066=DIRECTION('ref_axis',(0.,0.,-1.));
#7067=DIRECTION('center_axis',(0.,0.,1.));
#7068=DIRECTION('ref_axis',(1.,0.,0.));
#7069=DIRECTION('center_axis',(0.,-1.,0.));
#7070=DIRECTION('ref_axis',(0.,0.,-1.));
#7071=DIRECTION('center_axis',(0.,1.,0.));
#7072=DIRECTION('ref_axis',(1.,0.,0.));
#7073=DIRECTION('center_axis',(0.,-1.,0.));
#7074=DIRECTION('ref_axis',(1.,0.,0.));
#7075=DIRECTION('center_axis',(0.,-1.,0.));
#7076=DIRECTION('ref_axis',(0.,0.,-1.));
#7077=DIRECTION('center_axis',(6.12323399573676E-17,0.,1.));
#7078=DIRECTION('ref_axis',(1.,0.,0.));
#7079=DIRECTION('center_axis',(0.,-1.,0.));
#7080=DIRECTION('ref_axis',(0.,0.,-1.));
#7081=DIRECTION('center_axis',(0.,1.,0.));
#7082=DIRECTION('ref_axis',(1.,0.,0.));
#7083=DIRECTION('center_axis',(0.,-1.,0.));
#7084=DIRECTION('ref_axis',(1.,0.,0.));
#7085=DIRECTION('center_axis',(0.,-1.,0.));
#7086=DIRECTION('ref_axis',(0.,0.,-1.));
#7087=DIRECTION('center_axis',(0.,0.,1.));
#7088=DIRECTION('ref_axis',(1.,0.,0.));
#7089=DIRECTION('center_axis',(0.,-1.,0.));
#7090=DIRECTION('ref_axis',(0.,0.,-1.));
#7091=DIRECTION('center_axis',(0.,1.,0.));
#7092=DIRECTION('ref_axis',(1.,0.,0.));
#7093=DIRECTION('center_axis',(0.,1.,0.));
#7094=DIRECTION('ref_axis',(1.,0.,0.));
#7095=DIRECTION('',(0.,1.,0.));
#7096=DIRECTION('center_axis',(0.,-1.,0.));
#7097=DIRECTION('ref_axis',(1.,0.,0.));
#7098=DIRECTION('center_axis',(0.,-1.,0.));
#7099=DIRECTION('ref_axis',(1.,0.,0.));
#7100=DIRECTION('center_axis',(0.,1.,0.));
#7101=DIRECTION('ref_axis',(1.,0.,0.));
#7102=DIRECTION('center_axis',(0.,-1.,0.));
#7103=DIRECTION('ref_axis',(0.,0.,-1.));
#7104=DIRECTION('center_axis',(0.,0.,1.));
#7105=DIRECTION('ref_axis',(1.,0.,0.));
#7106=DIRECTION('center_axis',(0.,-1.,0.));
#7107=DIRECTION('ref_axis',(0.,0.,-1.));
#7108=DIRECTION('center_axis',(0.,-1.,0.));
#7109=DIRECTION('ref_axis',(-1.,0.,0.));
#7110=DIRECTION('center_axis',(0.,1.,0.));
#7111=DIRECTION('ref_axis',(1.,0.,0.));
#10456=CARTESIAN_POINT('',(0.,0.,0.));
#10457=CARTESIAN_POINT('Origin',(0.707106781186547,0.,0.707106781186548));
#10458=CARTESIAN_POINT('',(0.504455939115715,-0.04763,0.841298510752802));
#10459=CARTESIAN_POINT('',(0.841298510752802,-0.04763,0.504455939115715));
#10460=CARTESIAN_POINT('Ctrl Pts',(0.504455939115715,-0.04763,0.841298510752802));
#10461=CARTESIAN_POINT('Ctrl Pts',(0.508899795931835,-0.0740444353928835,
0.838633903678357));
#10462=CARTESIAN_POINT('Ctrl Pts',(0.517157748491652,-0.0999305678883309,
0.833661031856294));
#10463=CARTESIAN_POINT('Ctrl Pts',(0.537715343527944,-0.142345102874864,
0.820511285096538));
#10464=CARTESIAN_POINT('Ctrl Pts',(0.548874290046456,-0.159766064500479,
0.813159949759));
#10465=CARTESIAN_POINT('Ctrl Pts',(0.573915184558107,-0.190326085855194,
0.795684265985089));
#10466=CARTESIAN_POINT('Ctrl Pts',(0.587792702767295,-0.203463743702801,
0.78555112003688));
#10467=CARTESIAN_POINT('Ctrl Pts',(0.615966552324775,-0.224161999508995,
0.763642258217233));
#10468=CARTESIAN_POINT('Ctrl Pts',(0.631684198665438,-0.232861760990032,
0.750785745543687));
#10469=CARTESIAN_POINT('Ctrl Pts',(0.663382628119203,-0.244251601209411,
0.722929908501543));
#10470=CARTESIAN_POINT('Ctrl Pts',(0.679352081686668,-0.246942143572133,
0.707917883896095));
#10471=CARTESIAN_POINT('Ctrl Pts',(0.707917883896095,-0.246942143572133,
0.679352081686668));
#10472=CARTESIAN_POINT('Ctrl Pts',(0.722929908501543,-0.244251601209411,
0.663382628119203));
#10473=CARTESIAN_POINT('Ctrl Pts',(0.750785745543687,-0.232861760990032,
0.631684198665439));
#10474=CARTESIAN_POINT('Ctrl Pts',(0.763642258217232,-0.224161999508995,
0.615966552324775));
#10475=CARTESIAN_POINT('Ctrl Pts',(0.78555112003688,-0.203463743702801,
0.587792702767295));
#10476=CARTESIAN_POINT('Ctrl Pts',(0.795684265985088,-0.190326085855194,
0.573915184558108));
#10477=CARTESIAN_POINT('Ctrl Pts',(0.813159949759,-0.15976606450048,0.548874290046456));
#10478=CARTESIAN_POINT('Ctrl Pts',(0.820511285096538,-0.142345102874864,
0.537715343527944));
#10479=CARTESIAN_POINT('Ctrl Pts',(0.833661031856294,-0.099930567888331,
0.517157748491653));
#10480=CARTESIAN_POINT('Ctrl Pts',(0.838633903678357,-0.0740444353928835,
0.508899795931835));
#10481=CARTESIAN_POINT('Ctrl Pts',(0.841298510752801,-0.0476299999999999,
0.504455939115715));
#10482=CARTESIAN_POINT('',(0.528110872004958,-0.04763,0.871530771444223));
#10483=CARTESIAN_POINT('Origin',(0.707106781186547,-0.04763,0.707106781186548));
#10484=CARTESIAN_POINT('',(0.871530771444223,-0.04763,0.528110872004959));
#10485=CARTESIAN_POINT('Ctrl Pts',(0.871530771444223,-0.0476300000000001,
0.528110872004958));
#10486=CARTESIAN_POINT('Ctrl Pts',(0.87014664509073,-0.0609922781173483,
0.530395067942936));
#10487=CARTESIAN_POINT('Ctrl Pts',(0.868149331745851,-0.0742967091364493,
0.533674141594226));
#10488=CARTESIAN_POINT('Ctrl Pts',(0.85981294420286,-0.115492077056649,
0.54708917182331));
#10489=CARTESIAN_POINT('Ctrl Pts',(0.850993704737257,-0.141695629206859,
0.560922177770136));
#10490=CARTESIAN_POINT('Ctrl Pts',(0.830754510485543,-0.181890537957859,
0.590422647829571));
#10491=CARTESIAN_POINT('Ctrl Pts',(0.816896541396381,-0.201072148666545,
0.609616703125488));
#10492=CARTESIAN_POINT('Ctrl Pts',(0.792310597819928,-0.223955109275652,
0.641117951819998));
#10493=CARTESIAN_POINT('Ctrl Pts',(0.779109323683612,-0.232742381310829,
0.657208095763053));
#10494=CARTESIAN_POINT('Ctrl Pts',(0.750552691816206,-0.244234834628584,
0.68964083160521));
#10495=CARTESIAN_POINT('Ctrl Pts',(0.735185187071673,-0.246942143572133,
0.705971972091755));
#10496=CARTESIAN_POINT('Ctrl Pts',(0.705971972091754,-0.246942143572133,
0.735185187071673));
#10497=CARTESIAN_POINT('Ctrl Pts',(0.689640831605209,-0.244234834628584,
0.750552691816206));
#10498=CARTESIAN_POINT('Ctrl Pts',(0.657208095763052,-0.232742381310829,
0.779109323683612));
#10499=CARTESIAN_POINT('Ctrl Pts',(0.641117951819998,-0.223955109275652,
0.792310597819928));
#10500=CARTESIAN_POINT('Ctrl Pts',(0.609616703125487,-0.201072148666545,
0.816896541396382));
#10501=CARTESIAN_POINT('Ctrl Pts',(0.590422647829571,-0.181890537957858,
0.830754510485544));
#10502=CARTESIAN_POINT('Ctrl Pts',(0.560922177770135,-0.141695629206858,
0.850993704737257));
#10503=CARTESIAN_POINT('Ctrl Pts',(0.547089171823309,-0.115492077056649,
0.859812944202861));
#10504=CARTESIAN_POINT('Ctrl Pts',(0.533674141594226,-0.0742967091364491,
0.868149331745852));
#10505=CARTESIAN_POINT('Ctrl Pts',(0.530395067942936,-0.0609922781173483,
0.870146645090731));
#10506=CARTESIAN_POINT('Ctrl Pts',(0.528110872004958,-0.0476300000000001,
0.871530771444223));
#10507=CARTESIAN_POINT('Origin',(0.707106781186547,-0.04763,0.707106781186548));
#10508=CARTESIAN_POINT('Origin',(0.,-0.166705,0.));
#10509=CARTESIAN_POINT('',(0.242834539687906,-0.04763,0.989696097314));
#10510=CARTESIAN_POINT('Origin',(0.,-0.04763,0.));
#10511=CARTESIAN_POINT('',(-0.242834539687907,-0.04763,0.989696097314));
#10512=CARTESIAN_POINT('Ctrl Pts',(0.242834539687906,-0.04763,0.989696097314));
#10513=CARTESIAN_POINT('Ctrl Pts',(0.24024064412003,-0.0609922781173483,
0.990332542620729));
#10514=CARTESIAN_POINT('Ctrl Pts',(0.236509675094874,-0.0742967091364492,
0.991238884025248));
#10515=CARTESIAN_POINT('Ctrl Pts',(0.221129100087819,-0.115492077056649,
0.994830026707808));
#10516=CARTESIAN_POINT('Ctrl Pts',(0.205111543747588,-0.141695629206859,
0.998375294985966));
#10517=CARTESIAN_POINT('Ctrl Pts',(0.169940289819232,-0.181890537957859,
1.00492400591205));
#10518=CARTESIAN_POINT('Ctrl Pts',(0.1465689792446,-0.201072148666545,1.00869718865384));
#10519=CARTESIAN_POINT('Ctrl Pts',(0.106909345252087,-0.223955109275652,
1.01358704779679));
#10520=CARTESIAN_POINT('Ctrl Pts',(0.0861971848975941,-0.232742381310829,
1.0156297872271));
#10521=CARTESIAN_POINT('Ctrl Pts',(0.0430711894098822,-0.244234834628584,
1.01837060663223));
#10522=CARTESIAN_POINT('Ctrl Pts',(0.0206568624125605,-0.246942143572133,
1.019052));
#10523=CARTESIAN_POINT('Ctrl Pts',(-0.0206568624125608,-0.246942143572133,
1.019052));
#10524=CARTESIAN_POINT('Ctrl Pts',(-0.0430711894098825,-0.244234834628584,
1.01837060663223));
#10525=CARTESIAN_POINT('Ctrl Pts',(-0.0861971848975943,-0.232742381310829,
1.0156297872271));
#10526=CARTESIAN_POINT('Ctrl Pts',(-0.106909345252088,-0.223955109275652,
1.01358704779679));
#10527=CARTESIAN_POINT('Ctrl Pts',(-0.1465689792446,-0.201072148666545,
1.00869718865384));
#10528=CARTESIAN_POINT('Ctrl Pts',(-0.169940289819232,-0.181890537957859,
1.00492400591205));
#10529=CARTESIAN_POINT('Ctrl Pts',(-0.205111543747588,-0.141695629206859,
0.998375294985966));
#10530=CARTESIAN_POINT('Ctrl Pts',(-0.221129100087819,-0.115492077056649,
0.994830026707808));
#10531=CARTESIAN_POINT('Ctrl Pts',(-0.236509675094875,-0.0742967091364493,
0.991238884025248));
#10532=CARTESIAN_POINT('Ctrl Pts',(-0.24024064412003,-0.0609922781173483,
0.990332542620729));
#10533=CARTESIAN_POINT('Ctrl Pts',(-0.242834539687907,-0.04763,0.989696097314));
#10534=CARTESIAN_POINT('',(-0.528110872004959,-0.04763,0.871530771444223));
#10535=CARTESIAN_POINT('Origin',(0.,-0.04763,0.));
#10536=CARTESIAN_POINT('',(-0.871530771444223,-0.04763,0.528110872004958));
#10537=CARTESIAN_POINT('Ctrl Pts',(-0.528110872004958,-0.0476300000000001,
0.871530771444223));
#10538=CARTESIAN_POINT('Ctrl Pts',(-0.530395067942936,-0.0609922781173484,
0.87014664509073));
#10539=CARTESIAN_POINT('Ctrl Pts',(-0.533674141594226,-0.0742967091364493,
0.868149331745851));
#10540=CARTESIAN_POINT('Ctrl Pts',(-0.54708917182331,-0.115492077056649,
0.85981294420286));
#10541=CARTESIAN_POINT('Ctrl Pts',(-0.560922177770136,-0.141695629206859,
0.850993704737257));
#10542=CARTESIAN_POINT('Ctrl Pts',(-0.590422647829571,-0.181890537957859,
0.830754510485543));
#10543=CARTESIAN_POINT('Ctrl Pts',(-0.609616703125488,-0.201072148666545,
0.816896541396381));
#10544=CARTESIAN_POINT('Ctrl Pts',(-0.641117951819998,-0.223955109275652,
0.792310597819928));
#10545=CARTESIAN_POINT('Ctrl Pts',(-0.657208095763053,-0.232742381310829,
0.779109323683611));
#10546=CARTESIAN_POINT('Ctrl Pts',(-0.68964083160521,-0.244234834628584,
0.750552691816205));
#10547=CARTESIAN_POINT('Ctrl Pts',(-0.705971972091755,-0.246942143572133,
0.735185187071673));
#10548=CARTESIAN_POINT('Ctrl Pts',(-0.735185187071673,-0.246942143572133,
0.705971972091754));
#10549=CARTESIAN_POINT('Ctrl Pts',(-0.750552691816206,-0.244234834628584,
0.689640831605209));
#10550=CARTESIAN_POINT('Ctrl Pts',(-0.779109323683612,-0.232742381310829,
0.657208095763052));
#10551=CARTESIAN_POINT('Ctrl Pts',(-0.792310597819928,-0.223955109275652,
0.641117951819998));
#10552=CARTESIAN_POINT('Ctrl Pts',(-0.816896541396382,-0.201072148666545,
0.609616703125487));
#10553=CARTESIAN_POINT('Ctrl Pts',(-0.830754510485544,-0.181890537957858,
0.590422647829571));
#10554=CARTESIAN_POINT('Ctrl Pts',(-0.850993704737257,-0.141695629206858,
0.560922177770135));
#10555=CARTESIAN_POINT('Ctrl Pts',(-0.859812944202861,-0.115492077056649,
0.547089171823309));
#10556=CARTESIAN_POINT('Ctrl Pts',(-0.868149331745852,-0.0742967091364491,
0.533674141594226));
#10557=CARTESIAN_POINT('Ctrl Pts',(-0.870146645090731,-0.0609922781173483,
0.530395067942936));
#10558=CARTESIAN_POINT('Ctrl Pts',(-0.871530771444223,-0.04763,0.528110872004958));
#10559=CARTESIAN_POINT('',(-0.989696097314,-0.04763,0.242834539687906));
#10560=CARTESIAN_POINT('Origin',(0.,-0.04763,0.));
#10561=CARTESIAN_POINT('',(-1.019052,-0.246942143572133,1.248489836334E-16));
#10562=CARTESIAN_POINT('Ctrl Pts',(-0.989696097314,-0.04763,0.242834539687906));
#10563=CARTESIAN_POINT('Ctrl Pts',(-0.990332542620729,-0.0609922781173483,
0.24024064412003));
#10564=CARTESIAN_POINT('Ctrl Pts',(-0.991238884025248,-0.0742967091364492,
0.236509675094874));
#10565=CARTESIAN_POINT('Ctrl Pts',(-0.994830026707808,-0.115492077056649,
0.221129100087819));
#10566=CARTESIAN_POINT('Ctrl Pts',(-0.998375294985966,-0.141695629206859,
0.205111543747588));
#10567=CARTESIAN_POINT('Ctrl Pts',(-1.00492400591205,-0.181890537957859,
0.169940289819232));
#10568=CARTESIAN_POINT('Ctrl Pts',(-1.00869718865384,-0.201072148666545,
0.1465689792446));
#10569=CARTESIAN_POINT('Ctrl Pts',(-1.01358704779679,-0.223955109275652,
0.106909345252088));
#10570=CARTESIAN_POINT('Ctrl Pts',(-1.0156297872271,-0.232742381310829,
0.0861971848975944));
#10571=CARTESIAN_POINT('Ctrl Pts',(-1.01837060663223,-0.244234834628584,
0.0430711894098825));
#10572=CARTESIAN_POINT('Ctrl Pts',(-1.019052,-0.246942143572133,0.0206568624125608));
#10573=CARTESIAN_POINT('Ctrl Pts',(-1.019052,-0.246942143572133,1.2490009027033E-16));
#10574=CARTESIAN_POINT('',(-1.019052,-0.28578,1.24797876996471E-16));
#10575=CARTESIAN_POINT('',(-1.019052,-0.166705,1.24797876996471E-16));
#10576=CARTESIAN_POINT('Origin',(0.,-0.28578,0.));
#10577=CARTESIAN_POINT('',(-0.989696097314,-0.04763,-0.242834539687906));
#10578=CARTESIAN_POINT('Ctrl Pts',(-1.019052,-0.246942143572133,1.2490009027033E-16));
#10579=CARTESIAN_POINT('Ctrl Pts',(-1.019052,-0.246942143572133,-0.0206568624125605));
#10580=CARTESIAN_POINT('Ctrl Pts',(-1.01837060663223,-0.244234834628584,
-0.0430711894098822));
#10581=CARTESIAN_POINT('Ctrl Pts',(-1.0156297872271,-0.232742381310829,
-0.0861971848975941));
#10582=CARTESIAN_POINT('Ctrl Pts',(-1.01358704779679,-0.223955109275652,
-0.106909345252087));
#10583=CARTESIAN_POINT('Ctrl Pts',(-1.00869718865384,-0.201072148666546,
-0.1465689792446));
#10584=CARTESIAN_POINT('Ctrl Pts',(-1.00492400591205,-0.181890537957859,
-0.169940289819232));
#10585=CARTESIAN_POINT('Ctrl Pts',(-0.998375294985966,-0.141695629206859,
-0.205111543747588));
#10586=CARTESIAN_POINT('Ctrl Pts',(-0.994830026707808,-0.11549207705665,
-0.221129100087819));
#10587=CARTESIAN_POINT('Ctrl Pts',(-0.991238884025248,-0.0742967091364495,
-0.236509675094874));
#10588=CARTESIAN_POINT('Ctrl Pts',(-0.990332542620729,-0.0609922781173484,
-0.24024064412003));
#10589=CARTESIAN_POINT('Ctrl Pts',(-0.989696097314,-0.0476300000000001,
-0.242834539687907));
#10590=CARTESIAN_POINT('',(-0.871530771444223,-0.04763,-0.528110872004958));
#10591=CARTESIAN_POINT('Origin',(0.,-0.04763,0.));
#10592=CARTESIAN_POINT('',(-0.528110872004958,-0.04763,-0.871530771444223));
#10593=CARTESIAN_POINT('Ctrl Pts',(-0.871530771444223,-0.0476300000000001,
-0.528110872004958));
#10594=CARTESIAN_POINT('Ctrl Pts',(-0.87014664509073,-0.0609922781173484,
-0.530395067942936));
#10595=CARTESIAN_POINT('Ctrl Pts',(-0.868149331745851,-0.0742967091364494,
-0.533674141594226));
#10596=CARTESIAN_POINT('Ctrl Pts',(-0.85981294420286,-0.115492077056649,
-0.54708917182331));
#10597=CARTESIAN_POINT('Ctrl Pts',(-0.850993704737257,-0.141695629206859,
-0.560922177770136));
#10598=CARTESIAN_POINT('Ctrl Pts',(-0.830754510485543,-0.181890537957859,
-0.590422647829571));
#10599=CARTESIAN_POINT('Ctrl Pts',(-0.816896541396381,-0.201072148666546,
-0.609616703125488));
#10600=CARTESIAN_POINT('Ctrl Pts',(-0.792310597819928,-0.223955109275652,
-0.641117951819999));
#10601=CARTESIAN_POINT('Ctrl Pts',(-0.779109323683611,-0.232742381310829,
-0.657208095763053));
#10602=CARTESIAN_POINT('Ctrl Pts',(-0.750552691816205,-0.244234834628584,
-0.68964083160521));
#10603=CARTESIAN_POINT('Ctrl Pts',(-0.735185187071673,-0.246942143572133,
-0.705971972091755));
#10604=CARTESIAN_POINT('Ctrl Pts',(-0.705971972091754,-0.246942143572133,
-0.735185187071673));
#10605=CARTESIAN_POINT('Ctrl Pts',(-0.68964083160521,-0.244234834628584,
-0.750552691816206));
#10606=CARTESIAN_POINT('Ctrl Pts',(-0.657208095763052,-0.232742381310829,
-0.779109323683612));
#10607=CARTESIAN_POINT('Ctrl Pts',(-0.641117951819998,-0.223955109275652,
-0.792310597819928));
#10608=CARTESIAN_POINT('Ctrl Pts',(-0.609616703125488,-0.201072148666545,
-0.816896541396381));
#10609=CARTESIAN_POINT('Ctrl Pts',(-0.590422647829571,-0.181890537957859,
-0.830754510485543));
#10610=CARTESIAN_POINT('Ctrl Pts',(-0.560922177770136,-0.141695629206859,
-0.850993704737257));
#10611=CARTESIAN_POINT('Ctrl Pts',(-0.54708917182331,-0.115492077056649,
-0.85981294420286));
#10612=CARTESIAN_POINT('Ctrl Pts',(-0.533674141594226,-0.0742967091364494,
-0.868149331745852));
#10613=CARTESIAN_POINT('Ctrl Pts',(-0.530395067942936,-0.0609922781173484,
-0.870146645090731));
#10614=CARTESIAN_POINT('Ctrl Pts',(-0.528110872004958,-0.0476300000000001,
-0.871530771444223));
#10615=CARTESIAN_POINT('',(-0.242834539687906,-0.04763,-0.989696097314));
#10616=CARTESIAN_POINT('Origin',(0.,-0.04763,0.));
#10617=CARTESIAN_POINT('',(0.242834539687906,-0.04763,-0.989696097314));
#10618=CARTESIAN_POINT('Ctrl Pts',(-0.242834539687907,-0.04763,-0.989696097314));
#10619=CARTESIAN_POINT('Ctrl Pts',(-0.24024064412003,-0.0609922781173483,
-0.990332542620729));
#10620=CARTESIAN_POINT('Ctrl Pts',(-0.236509675094874,-0.0742967091364493,
-0.991238884025248));
#10621=CARTESIAN_POINT('Ctrl Pts',(-0.221129100087819,-0.115492077056649,
-0.994830026707808));
#10622=CARTESIAN_POINT('Ctrl Pts',(-0.205111543747588,-0.141695629206859,
-0.998375294985966));
#10623=CARTESIAN_POINT('Ctrl Pts',(-0.169940289819232,-0.181890537957859,
-1.00492400591205));
#10624=CARTESIAN_POINT('Ctrl Pts',(-0.1465689792446,-0.201072148666545,
-1.00869718865384));
#10625=CARTESIAN_POINT('Ctrl Pts',(-0.106909345252087,-0.223955109275652,
-1.01358704779679));
#10626=CARTESIAN_POINT('Ctrl Pts',(-0.0861971848975942,-0.232742381310829,
-1.0156297872271));
#10627=CARTESIAN_POINT('Ctrl Pts',(-0.0430711894098823,-0.244234834628584,
-1.01837060663223));
#10628=CARTESIAN_POINT('Ctrl Pts',(-0.0206568624125606,-0.246942143572133,
-1.019052));
#10629=CARTESIAN_POINT('Ctrl Pts',(0.0206568624125607,-0.246942143572133,
-1.019052));
#10630=CARTESIAN_POINT('Ctrl Pts',(0.0430711894098824,-0.244234834628584,
-1.01837060663223));
#10631=CARTESIAN_POINT('Ctrl Pts',(0.0861971848975943,-0.232742381310829,
-1.0156297872271));
#10632=CARTESIAN_POINT('Ctrl Pts',(0.106909345252088,-0.223955109275652,
-1.01358704779679));
#10633=CARTESIAN_POINT('Ctrl Pts',(0.1465689792446,-0.201072148666545,-1.00869718865384));
#10634=CARTESIAN_POINT('Ctrl Pts',(0.169940289819232,-0.181890537957859,
-1.00492400591205));
#10635=CARTESIAN_POINT('Ctrl Pts',(0.205111543747588,-0.141695629206859,
-0.998375294985966));
#10636=CARTESIAN_POINT('Ctrl Pts',(0.221129100087819,-0.115492077056649,
-0.994830026707808));
#10637=CARTESIAN_POINT('Ctrl Pts',(0.236509675094874,-0.0742967091364493,
-0.991238884025248));
#10638=CARTESIAN_POINT('Ctrl Pts',(0.24024064412003,-0.0609922781173484,
-0.990332542620729));
#10639=CARTESIAN_POINT('Ctrl Pts',(0.242834539687907,-0.04763,-0.989696097314));
#10640=CARTESIAN_POINT('',(0.528110872004958,-0.04763,-0.871530771444223));
#10641=CARTESIAN_POINT('Origin',(0.,-0.04763,0.));
#10642=CARTESIAN_POINT('',(0.871530771444223,-0.04763,-0.528110872004958));
#10643=CARTESIAN_POINT('Ctrl Pts',(0.528110872004958,-0.0476300000000001,
-0.871530771444223));
#10644=CARTESIAN_POINT('Ctrl Pts',(0.530395067942936,-0.0609922781173484,
-0.870146645090731));
#10645=CARTESIAN_POINT('Ctrl Pts',(0.533674141594226,-0.0742967091364493,
-0.868149331745851));
#10646=CARTESIAN_POINT('Ctrl Pts',(0.54708917182331,-0.115492077056649,
-0.85981294420286));
#10647=CARTESIAN_POINT('Ctrl Pts',(0.560922177770136,-0.141695629206859,
-0.850993704737257));
#10648=CARTESIAN_POINT('Ctrl Pts',(0.590422647829571,-0.181890537957859,
-0.830754510485543));
#10649=CARTESIAN_POINT('Ctrl Pts',(0.609616703125488,-0.201072148666545,
-0.816896541396381));
#10650=CARTESIAN_POINT('Ctrl Pts',(0.641117951819998,-0.223955109275652,
-0.792310597819928));
#10651=CARTESIAN_POINT('Ctrl Pts',(0.657208095763053,-0.232742381310829,
-0.779109323683612));
#10652=CARTESIAN_POINT('Ctrl Pts',(0.68964083160521,-0.244234834628584,
-0.750552691816206));
#10653=CARTESIAN_POINT('Ctrl Pts',(0.705971972091755,-0.246942143572133,
-0.735185187071673));
#10654=CARTESIAN_POINT('Ctrl Pts',(0.735185187071673,-0.246942143572133,
-0.705971972091754));
#10655=CARTESIAN_POINT('Ctrl Pts',(0.750552691816206,-0.244234834628584,
-0.68964083160521));
#10656=CARTESIAN_POINT('Ctrl Pts',(0.779109323683612,-0.232742381310829,
-0.657208095763053));
#10657=CARTESIAN_POINT('Ctrl Pts',(0.792310597819928,-0.223955109275652,
-0.641117951819998));
#10658=CARTESIAN_POINT('Ctrl Pts',(0.816896541396381,-0.201072148666545,
-0.609616703125488));
#10659=CARTESIAN_POINT('Ctrl Pts',(0.830754510485543,-0.181890537957859,
-0.590422647829571));
#10660=CARTESIAN_POINT('Ctrl Pts',(0.850993704737257,-0.141695629206859,
-0.560922177770136));
#10661=CARTESIAN_POINT('Ctrl Pts',(0.85981294420286,-0.115492077056649,
-0.54708917182331));
#10662=CARTESIAN_POINT('Ctrl Pts',(0.868149331745851,-0.0742967091364493,
-0.533674141594226));
#10663=CARTESIAN_POINT('Ctrl Pts',(0.870146645090731,-0.0609922781173484,
-0.530395067942936));
#10664=CARTESIAN_POINT('Ctrl Pts',(0.871530771444223,-0.0476300000000001,
-0.528110872004958));
#10665=CARTESIAN_POINT('',(0.989696097314,-0.04763,-0.242834539687906));
#10666=CARTESIAN_POINT('Origin',(0.,-0.04763,0.));
#10667=CARTESIAN_POINT('',(0.989696097314,-0.04763,0.242834539687906));
#10668=CARTESIAN_POINT('Ctrl Pts',(0.989696097314,-0.04763,-0.242834539687907));
#10669=CARTESIAN_POINT('Ctrl Pts',(0.990332542620729,-0.0609922781173483,
-0.24024064412003));
#10670=CARTESIAN_POINT('Ctrl Pts',(0.991238884025248,-0.0742967091364493,
-0.236509675094874));
#10671=CARTESIAN_POINT('Ctrl Pts',(0.994830026707808,-0.115492077056649,
-0.221129100087819));
#10672=CARTESIAN_POINT('Ctrl Pts',(0.998375294985966,-0.141695629206859,
-0.205111543747588));
#10673=CARTESIAN_POINT('Ctrl Pts',(1.00492400591205,-0.181890537957859,
-0.169940289819232));
#10674=CARTESIAN_POINT('Ctrl Pts',(1.00869718865384,-0.201072148666545,
-0.1465689792446));
#10675=CARTESIAN_POINT('Ctrl Pts',(1.01358704779679,-0.223955109275652,
-0.106909345252087));
#10676=CARTESIAN_POINT('Ctrl Pts',(1.0156297872271,-0.232742381310829,-0.0861971848975942));
#10677=CARTESIAN_POINT('Ctrl Pts',(1.01837060663223,-0.244234834628584,
-0.0430711894098823));
#10678=CARTESIAN_POINT('Ctrl Pts',(1.019052,-0.246942143572133,-0.0206568624125607));
#10679=CARTESIAN_POINT('Ctrl Pts',(1.019052,-0.246942143572133,0.0206568624125607));
#10680=CARTESIAN_POINT('Ctrl Pts',(1.01837060663223,-0.244234834628584,
0.0430711894098823));
#10681=CARTESIAN_POINT('Ctrl Pts',(1.0156297872271,-0.232742381310829,0.0861971848975942));
#10682=CARTESIAN_POINT('Ctrl Pts',(1.01358704779679,-0.223955109275652,
0.106909345252087));
#10683=CARTESIAN_POINT('Ctrl Pts',(1.00869718865384,-0.201072148666545,
0.1465689792446));
#10684=CARTESIAN_POINT('Ctrl Pts',(1.00492400591205,-0.181890537957859,
0.169940289819232));
#10685=CARTESIAN_POINT('Ctrl Pts',(0.998375294985966,-0.141695629206859,
0.205111543747588));
#10686=CARTESIAN_POINT('Ctrl Pts',(0.994830026707808,-0.115492077056649,
0.221129100087819));
#10687=CARTESIAN_POINT('Ctrl Pts',(0.991238884025248,-0.0742967091364492,
0.236509675094874));
#10688=CARTESIAN_POINT('Ctrl Pts',(0.990332542620729,-0.0609922781173483,
0.24024064412003));
#10689=CARTESIAN_POINT('Ctrl Pts',(0.989696097314,-0.04763,0.242834539687907));
#10690=CARTESIAN_POINT('Origin',(0.,-0.04763,0.));
#10691=CARTESIAN_POINT('Origin',(0.,-0.04763,0.));
#10692=CARTESIAN_POINT('',(0.238183666596899,-0.04763,0.951592097314));
#10693=CARTESIAN_POINT('Origin',(0.,-0.04763,0.));
#10694=CARTESIAN_POINT('Origin',(-1.94289029309402E-16,-0.04763,1.));
#10695=CARTESIAN_POINT('Origin',(-1.94289029309402E-16,0.,1.));
#10696=CARTESIAN_POINT('',(-0.2381836665969,-0.04763,0.951592097314));
#10697=CARTESIAN_POINT('Ctrl Pts',(-0.238183666596899,-0.0476299999999999,
0.951592097314));
#10698=CARTESIAN_POINT('Ctrl Pts',(-0.233157223576062,-0.0740444353928835,
0.952850216871763));
#10699=CARTESIAN_POINT('Ctrl Pts',(-0.223801617934946,-0.0999305678883309,
0.955173119738174));
#10700=CARTESIAN_POINT('Ctrl Pts',(-0.199966927975188,-0.142345102874864,
0.960411259488514));
#10701=CARTESIAN_POINT('Ctrl Pts',(-0.1868781821531,-0.159766064500479,
0.963103647174702));
#10702=CARTESIAN_POINT('Ctrl Pts',(-0.15681442133453,-0.190326085855194,
0.968453058988463));
#10703=CARTESIAN_POINT('Ctrl Pts',(-0.139836317888043,-0.203463743702801,
0.971100730005489));
#10704=CARTESIAN_POINT('Ctrl Pts',(-0.104422493053067,-0.224161999508995,
0.975530745318961));
#10705=CARTESIAN_POINT('Ctrl Pts',(-0.0842175114474176,-0.232861760990032,
0.977553872336861));
#10706=CARTESIAN_POINT('Ctrl Pts',(-0.0421062857595701,-0.244251601209411,
0.980270995488453));
#10707=CARTESIAN_POINT('Ctrl Pts',(-0.0201990724523197,-0.246942143572133,
0.980948));
#10708=CARTESIAN_POINT('Ctrl Pts',(0.020199072452319,-0.246942143572133,
0.980948));
#10709=CARTESIAN_POINT('Ctrl Pts',(0.0421062857595694,-0.244251601209411,
0.980270995488454));
#10710=CARTESIAN_POINT('Ctrl Pts',(0.0842175114474169,-0.232861760990032,
0.977553872336861));
#10711=CARTESIAN_POINT('Ctrl Pts',(0.104422493053067,-0.224161999508995,
0.975530745318961));
#10712=CARTESIAN_POINT('Ctrl Pts',(0.139836317888042,-0.203463743702801,
0.971100730005489));
#10713=CARTESIAN_POINT('Ctrl Pts',(0.15681442133453,-0.190326085855194,
0.968453058988463));
#10714=CARTESIAN_POINT('Ctrl Pts',(0.1868781821531,-0.15976606450048,0.963103647174702));
#10715=CARTESIAN_POINT('Ctrl Pts',(0.199966927975188,-0.142345102874864,
0.960411259488514));
#10716=CARTESIAN_POINT('Ctrl Pts',(0.223801617934945,-0.0999305678883309,
0.955173119738174));
#10717=CARTESIAN_POINT('Ctrl Pts',(0.233157223576061,-0.0740444353928835,
0.952850216871763));
#10718=CARTESIAN_POINT('Ctrl Pts',(0.238183666596899,-0.0476299999999999,
0.951592097314));
#10719=CARTESIAN_POINT('Origin',(-1.94289029309402E-16,-0.04763,1.));
#10720=CARTESIAN_POINT('Origin',(0.,-0.04763,0.));
#10721=CARTESIAN_POINT('',(-0.504455939115715,-0.04763,0.841298510752802));
#10722=CARTESIAN_POINT('Origin',(0.,-0.04763,0.));
#10723=CARTESIAN_POINT('Origin',(-0.707106781186548,-0.04763,0.707106781186547));
#10724=CARTESIAN_POINT('Origin',(-0.707106781186548,0.,0.707106781186547));
#10725=CARTESIAN_POINT('',(-0.841298510752802,-0.04763,0.504455939115715));
#10726=CARTESIAN_POINT('Ctrl Pts',(-0.841298510752802,-0.04763,0.504455939115715));
#10727=CARTESIAN_POINT('Ctrl Pts',(-0.838633903678357,-0.0740444353928835,
0.508899795931835));
#10728=CARTESIAN_POINT('Ctrl Pts',(-0.833661031856294,-0.0999305678883309,
0.517157748491652));
#10729=CARTESIAN_POINT('Ctrl Pts',(-0.820511285096538,-0.142345102874864,
0.537715343527944));
#10730=CARTESIAN_POINT('Ctrl Pts',(-0.813159949759,-0.159766064500479,0.548874290046456));
#10731=CARTESIAN_POINT('Ctrl Pts',(-0.795684265985089,-0.190326085855194,
0.573915184558107));
#10732=CARTESIAN_POINT('Ctrl Pts',(-0.78555112003688,-0.203463743702801,
0.587792702767295));
#10733=CARTESIAN_POINT('Ctrl Pts',(-0.763642258217233,-0.224161999508995,
0.615966552324775));
#10734=CARTESIAN_POINT('Ctrl Pts',(-0.750785745543687,-0.232861760990032,
0.631684198665438));
#10735=CARTESIAN_POINT('Ctrl Pts',(-0.722929908501543,-0.244251601209411,
0.663382628119203));
#10736=CARTESIAN_POINT('Ctrl Pts',(-0.707917883896095,-0.246942143572133,
0.679352081686668));
#10737=CARTESIAN_POINT('Ctrl Pts',(-0.679352081686668,-0.246942143572133,
0.707917883896095));
#10738=CARTESIAN_POINT('Ctrl Pts',(-0.663382628119203,-0.244251601209411,
0.722929908501544));
#10739=CARTESIAN_POINT('Ctrl Pts',(-0.631684198665438,-0.232861760990031,
0.750785745543687));
#10740=CARTESIAN_POINT('Ctrl Pts',(-0.615966552324775,-0.224161999508995,
0.763642258217233));
#10741=CARTESIAN_POINT('Ctrl Pts',(-0.587792702767295,-0.203463743702801,
0.78555112003688));
#10742=CARTESIAN_POINT('Ctrl Pts',(-0.573915184558107,-0.190326085855194,
0.795684265985088));
#10743=CARTESIAN_POINT('Ctrl Pts',(-0.548874290046456,-0.159766064500479,
0.813159949759));
#10744=CARTESIAN_POINT('Ctrl Pts',(-0.537715343527944,-0.142345102874864,
0.820511285096538));
#10745=CARTESIAN_POINT('Ctrl Pts',(-0.517157748491652,-0.0999305678883309,
0.833661031856294));
#10746=CARTESIAN_POINT('Ctrl Pts',(-0.508899795931835,-0.0740444353928835,
0.838633903678357));
#10747=CARTESIAN_POINT('Ctrl Pts',(-0.504455939115716,-0.04763,0.841298510752801));
#10748=CARTESIAN_POINT('Origin',(-0.707106781186548,-0.04763,0.707106781186547));
#10749=CARTESIAN_POINT('Origin',(0.,-0.04763,0.));
#10750=CARTESIAN_POINT('',(-0.951592097314,-0.04763,0.238183666596899));
#10751=CARTESIAN_POINT('Origin',(0.,-0.04763,0.));
#10752=CARTESIAN_POINT('Origin',(-1.,-0.04763,-1.11022302462516E-16));
#10753=CARTESIAN_POINT('Origin',(-1.,0.,-1.11022302462516E-16));
#10754=CARTESIAN_POINT('',(-0.951592097314,-0.04763,-0.2381836665969));
#10755=CARTESIAN_POINT('',(-0.980948,-0.246942143572133,1.08514323328844E-18));
#10756=CARTESIAN_POINT('Ctrl Pts',(-0.951592097314,-0.04763,-0.238183666596899));
#10757=CARTESIAN_POINT('Ctrl Pts',(-0.952850216871763,-0.0740444353928835,
-0.233157223576062));
#10758=CARTESIAN_POINT('Ctrl Pts',(-0.955173119738174,-0.0999305678883309,
-0.223801617934946));
#10759=CARTESIAN_POINT('Ctrl Pts',(-0.960411259488514,-0.142345102874864,
-0.199966927975188));
#10760=CARTESIAN_POINT('Ctrl Pts',(-0.963103647174702,-0.159766064500479,
-0.1868781821531));
#10761=CARTESIAN_POINT('Ctrl Pts',(-0.968453058988463,-0.190326085855194,
-0.15681442133453));
#10762=CARTESIAN_POINT('Ctrl Pts',(-0.971100730005489,-0.203463743702801,
-0.139836317888043));
#10763=CARTESIAN_POINT('Ctrl Pts',(-0.975530745318961,-0.224161999508995,
-0.104422493053067));
#10764=CARTESIAN_POINT('Ctrl Pts',(-0.977553872336861,-0.232861760990032,
-0.0842175114474175));
#10765=CARTESIAN_POINT('Ctrl Pts',(-0.980270995488453,-0.244251601209411,
-0.0421062857595699));
#10766=CARTESIAN_POINT('Ctrl Pts',(-0.980948,-0.246942143572133,-0.0201990724523195));
#10767=CARTESIAN_POINT('Ctrl Pts',(-0.980948,-0.246942143572133,-1.17961196366423E-16));
#10768=CARTESIAN_POINT('Origin',(-1.,-0.04763,-1.11022302462516E-16));
#10769=CARTESIAN_POINT('Ctrl Pts',(-0.980948,-0.246942143572133,-1.17961196366423E-16));
#10770=CARTESIAN_POINT('Ctrl Pts',(-0.980948,-0.246942143572133,0.0201990724523192));
#10771=CARTESIAN_POINT('Ctrl Pts',(-0.980270995488453,-0.244251601209411,
0.0421062857595695));
#10772=CARTESIAN_POINT('Ctrl Pts',(-0.977553872336861,-0.232861760990032,
0.0842175114474169));
#10773=CARTESIAN_POINT('Ctrl Pts',(-0.975530745318961,-0.224161999508995,
0.104422493053066));
#10774=CARTESIAN_POINT('Ctrl Pts',(-0.971100730005489,-0.203463743702801,
0.139836317888042));
#10775=CARTESIAN_POINT('Ctrl Pts',(-0.968453058988463,-0.190326085855194,
0.15681442133453));
#10776=CARTESIAN_POINT('Ctrl Pts',(-0.963103647174702,-0.15976606450048,
0.1868781821531));
#10777=CARTESIAN_POINT('Ctrl Pts',(-0.960411259488514,-0.142345102874864,
0.199966927975188));
#10778=CARTESIAN_POINT('Ctrl Pts',(-0.955173119738174,-0.099930567888331,
0.223801617934945));
#10779=CARTESIAN_POINT('Ctrl Pts',(-0.952850216871763,-0.0740444353928835,
0.233157223576061));
#10780=CARTESIAN_POINT('Ctrl Pts',(-0.951592097314,-0.04763,0.238183666596899));
#10781=CARTESIAN_POINT('Origin',(0.,-0.04763,0.));
#10782=CARTESIAN_POINT('',(-0.841298510752802,-0.04763,-0.504455939115715));
#10783=CARTESIAN_POINT('Origin',(0.,-0.04763,0.));
#10784=CARTESIAN_POINT('Origin',(-0.707106781186547,-0.04763,-0.707106781186548));
#10785=CARTESIAN_POINT('Origin',(-0.707106781186547,0.,-0.707106781186548));
#10786=CARTESIAN_POINT('',(-0.504455939115715,-0.04763,-0.841298510752802));
#10787=CARTESIAN_POINT('Ctrl Pts',(-0.504455939115715,-0.04763,-0.841298510752802));
#10788=CARTESIAN_POINT('Ctrl Pts',(-0.508899795931835,-0.0740444353928835,
-0.838633903678357));
#10789=CARTESIAN_POINT('Ctrl Pts',(-0.517157748491652,-0.0999305678883309,
-0.833661031856294));
#10790=CARTESIAN_POINT('Ctrl Pts',(-0.537715343527944,-0.142345102874864,
-0.820511285096538));
#10791=CARTESIAN_POINT('Ctrl Pts',(-0.548874290046456,-0.159766064500479,
-0.813159949759));
#10792=CARTESIAN_POINT('Ctrl Pts',(-0.573915184558107,-0.190326085855194,
-0.795684265985089));
#10793=CARTESIAN_POINT('Ctrl Pts',(-0.587792702767295,-0.203463743702801,
-0.78555112003688));
#10794=CARTESIAN_POINT('Ctrl Pts',(-0.615966552324775,-0.224161999508995,
-0.763642258217233));
#10795=CARTESIAN_POINT('Ctrl Pts',(-0.631684198665438,-0.232861760990032,
-0.750785745543687));
#10796=CARTESIAN_POINT('Ctrl Pts',(-0.663382628119203,-0.244251601209411,
-0.722929908501543));
#10797=CARTESIAN_POINT('Ctrl Pts',(-0.679352081686668,-0.246942143572133,
-0.707917883896095));
#10798=CARTESIAN_POINT('Ctrl Pts',(-0.707917883896095,-0.246942143572133,
-0.679352081686668));
#10799=CARTESIAN_POINT('Ctrl Pts',(-0.722929908501543,-0.244251601209411,
-0.663382628119203));
#10800=CARTESIAN_POINT('Ctrl Pts',(-0.750785745543687,-0.232861760990032,
-0.631684198665439));
#10801=CARTESIAN_POINT('Ctrl Pts',(-0.763642258217232,-0.224161999508995,
-0.615966552324775));
#10802=CARTESIAN_POINT('Ctrl Pts',(-0.78555112003688,-0.203463743702801,
-0.587792702767295));
#10803=CARTESIAN_POINT('Ctrl Pts',(-0.795684265985088,-0.190326085855194,
-0.573915184558107));
#10804=CARTESIAN_POINT('Ctrl Pts',(-0.813159949759,-0.15976606450048,-0.548874290046456));
#10805=CARTESIAN_POINT('Ctrl Pts',(-0.820511285096538,-0.142345102874864,
-0.537715343527944));
#10806=CARTESIAN_POINT('Ctrl Pts',(-0.833661031856294,-0.0999305678883311,
-0.517157748491652));
#10807=CARTESIAN_POINT('Ctrl Pts',(-0.838633903678357,-0.0740444353928836,
-0.508899795931835));
#10808=CARTESIAN_POINT('Ctrl Pts',(-0.841298510752801,-0.04763,-0.504455939115715));
#10809=CARTESIAN_POINT('Origin',(-0.707106781186547,-0.04763,-0.707106781186548));
#10810=CARTESIAN_POINT('Origin',(0.,-0.04763,0.));
#10811=CARTESIAN_POINT('',(-0.238183666596899,-0.04763,-0.951592097314));
#10812=CARTESIAN_POINT('Origin',(0.,-0.04763,0.));
#10813=CARTESIAN_POINT('Origin',(5.55111512312578E-17,-0.04763,-1.));
#10814=CARTESIAN_POINT('Origin',(5.55111512312578E-17,0.,-1.));
#10815=CARTESIAN_POINT('',(0.238183666596899,-0.04763,-0.951592097314));
#10816=CARTESIAN_POINT('Ctrl Pts',(0.238183666596899,-0.04763,-0.951592097314));
#10817=CARTESIAN_POINT('Ctrl Pts',(0.233157223576062,-0.0740444353928835,
-0.952850216871763));
#10818=CARTESIAN_POINT('Ctrl Pts',(0.223801617934946,-0.099930567888331,
-0.955173119738174));
#10819=CARTESIAN_POINT('Ctrl Pts',(0.199966927975188,-0.142345102874864,
-0.960411259488514));
#10820=CARTESIAN_POINT('Ctrl Pts',(0.1868781821531,-0.15976606450048,-0.963103647174702));
#10821=CARTESIAN_POINT('Ctrl Pts',(0.15681442133453,-0.190326085855194,
-0.968453058988463));
#10822=CARTESIAN_POINT('Ctrl Pts',(0.139836317888042,-0.203463743702801,
-0.971100730005489));
#10823=CARTESIAN_POINT('Ctrl Pts',(0.104422493053067,-0.224161999508995,
-0.975530745318961));
#10824=CARTESIAN_POINT('Ctrl Pts',(0.0842175114474173,-0.232861760990032,
-0.977553872336861));
#10825=CARTESIAN_POINT('Ctrl Pts',(0.0421062857595698,-0.244251601209411,
-0.980270995488453));
#10826=CARTESIAN_POINT('Ctrl Pts',(0.0201990724523194,-0.246942143572133,
-0.980948));
#10827=CARTESIAN_POINT('Ctrl Pts',(-0.0201990724523193,-0.246942143572133,
-0.980948));
#10828=CARTESIAN_POINT('Ctrl Pts',(-0.0421062857595697,-0.244251601209411,
-0.980270995488453));
#10829=CARTESIAN_POINT('Ctrl Pts',(-0.0842175114474171,-0.232861760990032,
-0.977553872336861));
#10830=CARTESIAN_POINT('Ctrl Pts',(-0.104422493053067,-0.224161999508995,
-0.975530745318961));
#10831=CARTESIAN_POINT('Ctrl Pts',(-0.139836317888042,-0.203463743702801,
-0.971100730005489));
#10832=CARTESIAN_POINT('Ctrl Pts',(-0.15681442133453,-0.190326085855194,
-0.968453058988463));
#10833=CARTESIAN_POINT('Ctrl Pts',(-0.1868781821531,-0.15976606450048,-0.963103647174702));
#10834=CARTESIAN_POINT('Ctrl Pts',(-0.199966927975188,-0.142345102874864,
-0.960411259488514));
#10835=CARTESIAN_POINT('Ctrl Pts',(-0.223801617934945,-0.099930567888331,
-0.955173119738174));
#10836=CARTESIAN_POINT('Ctrl Pts',(-0.233157223576062,-0.0740444353928835,
-0.952850216871763));
#10837=CARTESIAN_POINT('Ctrl Pts',(-0.238183666596899,-0.0476299999999999,
-0.951592097314));
#10838=CARTESIAN_POINT('Origin',(5.55111512312578E-17,-0.04763,-1.));
#10839=CARTESIAN_POINT('Origin',(0.,-0.04763,0.));
#10840=CARTESIAN_POINT('',(0.504455939115715,-0.04763,-0.841298510752802));
#10841=CARTESIAN_POINT('Origin',(0.,-0.04763,0.));
#10842=CARTESIAN_POINT('Origin',(0.707106781186548,-0.04763,-0.707106781186547));
#10843=CARTESIAN_POINT('Origin',(0.707106781186548,0.,-0.707106781186547));
#10844=CARTESIAN_POINT('',(0.841298510752802,-0.04763,-0.504455939115715));
#10845=CARTESIAN_POINT('Ctrl Pts',(0.841298510752802,-0.04763,-0.504455939115715));
#10846=CARTESIAN_POINT('Ctrl Pts',(0.838633903678357,-0.0740444353928835,
-0.508899795931835));
#10847=CARTESIAN_POINT('Ctrl Pts',(0.833661031856294,-0.0999305678883309,
-0.517157748491652));
#10848=CARTESIAN_POINT('Ctrl Pts',(0.820511285096538,-0.142345102874864,
-0.537715343527944));
#10849=CARTESIAN_POINT('Ctrl Pts',(0.813159949759,-0.159766064500479,-0.548874290046456));
#10850=CARTESIAN_POINT('Ctrl Pts',(0.795684265985088,-0.190326085855194,
-0.573915184558107));
#10851=CARTESIAN_POINT('Ctrl Pts',(0.78555112003688,-0.203463743702801,
-0.587792702767295));
#10852=CARTESIAN_POINT('Ctrl Pts',(0.763642258217233,-0.224161999508995,
-0.615966552324775));
#10853=CARTESIAN_POINT('Ctrl Pts',(0.750785745543687,-0.232861760990032,
-0.631684198665438));
#10854=CARTESIAN_POINT('Ctrl Pts',(0.722929908501543,-0.244251601209411,
-0.663382628119203));
#10855=CARTESIAN_POINT('Ctrl Pts',(0.707917883896095,-0.246942143572133,
-0.679352081686668));
#10856=CARTESIAN_POINT('Ctrl Pts',(0.679352081686668,-0.246942143572133,
-0.707917883896095));
#10857=CARTESIAN_POINT('Ctrl Pts',(0.663382628119203,-0.244251601209411,
-0.722929908501543));
#10858=CARTESIAN_POINT('Ctrl Pts',(0.631684198665438,-0.232861760990032,
-0.750785745543687));
#10859=CARTESIAN_POINT('Ctrl Pts',(0.615966552324775,-0.224161999508995,
-0.763642258217232));
#10860=CARTESIAN_POINT('Ctrl Pts',(0.587792702767295,-0.203463743702801,
-0.78555112003688));
#10861=CARTESIAN_POINT('Ctrl Pts',(0.573915184558107,-0.190326085855194,
-0.795684265985088));
#10862=CARTESIAN_POINT('Ctrl Pts',(0.548874290046456,-0.159766064500479,
-0.813159949759));
#10863=CARTESIAN_POINT('Ctrl Pts',(0.537715343527944,-0.142345102874864,
-0.820511285096538));
#10864=CARTESIAN_POINT('Ctrl Pts',(0.517157748491652,-0.099930567888331,
-0.833661031856294));
#10865=CARTESIAN_POINT('Ctrl Pts',(0.508899795931835,-0.0740444353928835,
-0.838633903678357));
#10866=CARTESIAN_POINT('Ctrl Pts',(0.504455939115715,-0.04763,-0.841298510752801));
#10867=CARTESIAN_POINT('Origin',(0.707106781186548,-0.04763,-0.707106781186547));
#10868=CARTESIAN_POINT('Origin',(0.,-0.166705,0.));
#10869=CARTESIAN_POINT('',(-0.980948,-0.28578,1.20131482833E-16));
#10870=CARTESIAN_POINT('Origin',(0.,-0.28578,0.));
#10871=CARTESIAN_POINT('',(-0.980948,-0.166705,1.20131482833E-16));
#10872=CARTESIAN_POINT('',(0.951592097314,-0.04763,0.238183666596899));
#10873=CARTESIAN_POINT('Origin',(0.,-0.04763,0.));
#10874=CARTESIAN_POINT('',(0.951592097314,-0.04763,-0.238183666596899));
#10875=CARTESIAN_POINT('Ctrl Pts',(0.951592097314,-0.04763,0.238183666596899));
#10876=CARTESIAN_POINT('Ctrl Pts',(0.952850216871763,-0.0740444353928835,
0.233157223576062));
#10877=CARTESIAN_POINT('Ctrl Pts',(0.955173119738174,-0.099930567888331,
0.223801617934945));
#10878=CARTESIAN_POINT('Ctrl Pts',(0.960411259488514,-0.142345102874864,
0.199966927975188));
#10879=CARTESIAN_POINT('Ctrl Pts',(0.963103647174702,-0.15976606450048,
0.1868781821531));
#10880=CARTESIAN_POINT('Ctrl Pts',(0.968453058988463,-0.190326085855194,
0.15681442133453));
#10881=CARTESIAN_POINT('Ctrl Pts',(0.971100730005489,-0.203463743702801,
0.139836317888042));
#10882=CARTESIAN_POINT('Ctrl Pts',(0.975530745318961,-0.224161999508995,
0.104422493053067));
#10883=CARTESIAN_POINT('Ctrl Pts',(0.977553872336861,-0.232861760990032,
0.0842175114474172));
#10884=CARTESIAN_POINT('Ctrl Pts',(0.980270995488453,-0.244251601209411,
0.0421062857595697));
#10885=CARTESIAN_POINT('Ctrl Pts',(0.980948,-0.246942143572133,0.0201990724523194));
#10886=CARTESIAN_POINT('Ctrl Pts',(0.980948,-0.246942143572133,-0.0201990724523194));
#10887=CARTESIAN_POINT('Ctrl Pts',(0.980270995488453,-0.244251601209411,
-0.0421062857595697));
#10888=CARTESIAN_POINT('Ctrl Pts',(0.977553872336861,-0.232861760990032,
-0.0842175114474172));
#10889=CARTESIAN_POINT('Ctrl Pts',(0.975530745318961,-0.224161999508995,
-0.104422493053067));
#10890=CARTESIAN_POINT('Ctrl Pts',(0.971100730005489,-0.203463743702801,
-0.139836317888042));
#10891=CARTESIAN_POINT('Ctrl Pts',(0.968453058988463,-0.190326085855194,
-0.15681442133453));
#10892=CARTESIAN_POINT('Ctrl Pts',(0.963103647174702,-0.15976606450048,
-0.1868781821531));
#10893=CARTESIAN_POINT('Ctrl Pts',(0.960411259488514,-0.142345102874864,
-0.199966927975188));
#10894=CARTESIAN_POINT('Ctrl Pts',(0.955173119738174,-0.099930567888331,
-0.223801617934945));
#10895=CARTESIAN_POINT('Ctrl Pts',(0.952850216871763,-0.0740444353928835,
-0.233157223576062));
#10896=CARTESIAN_POINT('Ctrl Pts',(0.951592097314,-0.0476299999999999,-0.238183666596899));
#10897=CARTESIAN_POINT('Origin',(0.,-0.04763,0.));
#10898=CARTESIAN_POINT('Origin',(0.,-0.04763,0.));
#10899=CARTESIAN_POINT('Origin',(1.,-0.04763,0.));
#10900=CARTESIAN_POINT('Origin',(1.,0.,0.));
#10901=CARTESIAN_POINT('Origin',(1.,-0.04763,0.));
#10902=CARTESIAN_POINT('Origin',(0.,-0.28578,0.));
#10903=CARTESIAN_POINT('Origin',(0.,-0.04763,0.));
#11000=UNCERTAINTY_MEASURE_WITH_UNIT(LENGTH_MEASURE(0.001),#11036,
'DISTANCE_ACCURACY_VALUE',
'Maximum model space distance between geometric entities at asserted c
onnectivities');
#11002=UNCERTAINTY_MEASURE_WITH_UNIT(LENGTH_MEASURE(0.001),#11036,
'DISTANCE_ACCURACY_VALUE',
'Maximum model space distance between geometric entities at asserted c
onnectivities');
#11033=(
GEOMETRIC_REPRESENTATION_CONTEXT(3)
GLOBAL_UNCERTAINTY_ASSIGNED_CONTEXT((#11000))
GLOBAL_UNIT_ASSIGNED_CONTEXT((#11036,#11038,#11039))
REPRESENTATION_CONTEXT('','3D')
);
#11035=(
GEOMETRIC_REPRESENTATION_CONTEXT(3)
GLOBAL_UNCERTAINTY_ASSIGNED_CONTEXT((#11002))
GLOBAL_UNIT_ASSIGNED_CONTEXT((#11036,#11038,#11039))
REPRESENTATION_CONTEXT('','3D')
);
#11036=(
LENGTH_UNIT()
NAMED_UNIT(*)
SI_UNIT(.CENTI.,.METRE.)
);
#11038=(
NAMED_UNIT(*)
PLANE_ANGLE_UNIT()
SI_UNIT($,.RADIAN.)
);
#11039=(
NAMED_UNIT(*)
SI_UNIT($,.STERADIAN.)
SOLID_ANGLE_UNIT()
);
#11070=SHAPE_DEFINITION_REPRESENTATION(#11114,#11183);
#11114=PRODUCT_DEFINITION_SHAPE('',$,#11216);
#11183=SHAPE_REPRESENTATION('',(#5560),#11033);
#11185=PRODUCT_DEFINITION_CONTEXT('part definition',#11283,'design');
#11216=PRODUCT_DEFINITION('Cage','Cage',#11248,#11185);
#11248=PRODUCT_DEFINITION_FORMATION('',$,#11315);
#11283=APPLICATION_CONTEXT(
'Core Data for Automotive Mechanical Design Process');
#11284=PRODUCT_CONTEXT('part definition',#11283,'mechanical');
#11315=PRODUCT('Cage','Cage','Cage',(#11284));
#11380=COLOUR_RGB('Grey',0.48,0.52,0.57);
#11381=FILL_AREA_STYLE_COLOUR('',#11380);
#11382=FILL_AREA_STYLE('',(#11381));
#11383=SURFACE_STYLE_FILL_AREA(#11382);
#11384=SURFACE_SIDE_STYLE('',(#11383));
#11385=SURFACE_STYLE_USAGE(.BOTH.,#11384);
#11386=PRESENTATION_STYLE_ASSIGNMENT((#11385));
ENDSEC;
END-ISO-10303-21;
